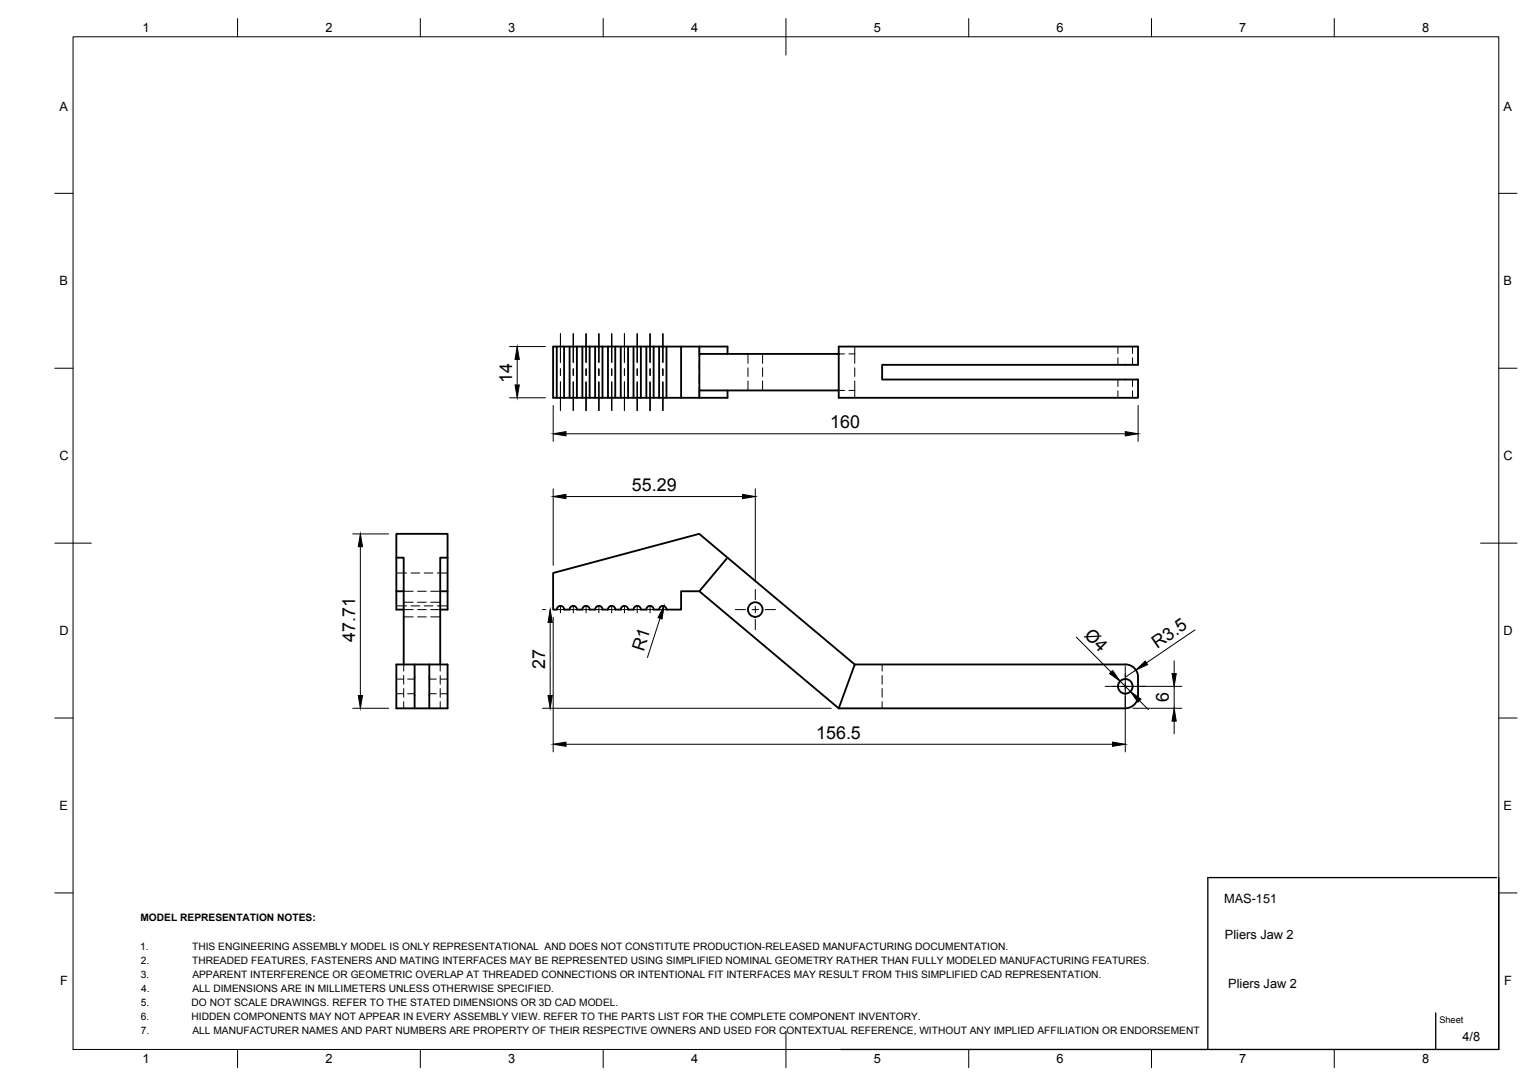
ISO-10303-21;
HEADER;
/* Generated by software containing ST-Developer
 * from STEP Tools, Inc. (www.steptools.com) 
 */

FILE_DESCRIPTION(
/* description */ ('STEP AP214'),
/* implementation_level */ '2;1');

FILE_NAME(
/* name */ 'Pliers Jaw 2.step',
/* time_stamp */ '2026-11-04T19:14:12-08:00',
/* author */ (''),
/* organization */ (''),
/* preprocessor_version */ 'ST-DEVELOPER v20.2',
/* originating_system */ 'Autodesk Translation Framework v15.17.0.0',
/* authorisation */ '');

FILE_SCHEMA (('AUTOMOTIVE_DESIGN { 1 0 10303 214 3 1 1 }'));
ENDSEC;

DATA;
#10=MECHANICAL_DESIGN_GEOMETRIC_PRESENTATION_REPRESENTATION('',(#100),#5990);
#86=SHAPE_REPRESENTATION_RELATIONSHIP('SRR','None',#6022,#93);
#93=ADVANCED_BREP_SHAPE_REPRESENTATION('',(#107),#5984);
#100=STYLED_ITEM('',(#6065),#107);
#107=MANIFOLD_SOLID_BREP('Body1',#3270);
#121=FACE_BOUND('',#479,.T.);
#122=FACE_BOUND('',#484,.T.);
#123=FACE_BOUND('',#516,.T.);
#124=FACE_BOUND('',#520,.T.);
#125=FACE_BOUND('',#522,.T.);
#126=FACE_BOUND('',#524,.T.);
#167=PLANE('',#3447);
#168=PLANE('',#3450);
#169=PLANE('',#3451);
#170=PLANE('',#3452);
#171=PLANE('',#3462);
#172=PLANE('',#3465);
#173=PLANE('',#3466);
#174=PLANE('',#3476);
#175=PLANE('',#3477);
#176=PLANE('',#3478);
#177=PLANE('',#3479);
#178=PLANE('',#3480);
#179=PLANE('',#3481);
#180=PLANE('',#3482);
#181=PLANE('',#3483);
#182=PLANE('',#3484);
#183=PLANE('',#3485);
#184=PLANE('',#3486);
#185=PLANE('',#3487);
#186=PLANE('',#3488);
#187=PLANE('',#3489);
#188=PLANE('',#3490);
#189=PLANE('',#3491);
#190=PLANE('',#3492);
#191=PLANE('',#3502);
#192=PLANE('',#3503);
#193=PLANE('',#3504);
#194=PLANE('',#3505);
#195=PLANE('',#3506);
#196=PLANE('',#3507);
#197=PLANE('',#3508);
#198=PLANE('',#3511);
#199=PLANE('',#3514);
#289=FACE_OUTER_BOUND('',#475,.T.);
#290=FACE_OUTER_BOUND('',#476,.T.);
#291=FACE_OUTER_BOUND('',#477,.T.);
#292=FACE_OUTER_BOUND('',#478,.T.);
#293=FACE_OUTER_BOUND('',#480,.T.);
#294=FACE_OUTER_BOUND('',#481,.T.);
#295=FACE_OUTER_BOUND('',#482,.T.);
#296=FACE_OUTER_BOUND('',#483,.T.);
#297=FACE_OUTER_BOUND('',#485,.T.);
#298=FACE_OUTER_BOUND('',#486,.T.);
#299=FACE_OUTER_BOUND('',#487,.T.);
#300=FACE_OUTER_BOUND('',#488,.T.);
#301=FACE_OUTER_BOUND('',#489,.T.);
#302=FACE_OUTER_BOUND('',#490,.T.);
#303=FACE_OUTER_BOUND('',#491,.T.);
#304=FACE_OUTER_BOUND('',#492,.T.);
#305=FACE_OUTER_BOUND('',#493,.T.);
#306=FACE_OUTER_BOUND('',#494,.T.);
#307=FACE_OUTER_BOUND('',#495,.T.);
#308=FACE_OUTER_BOUND('',#496,.T.);
#309=FACE_OUTER_BOUND('',#497,.T.);
#310=FACE_OUTER_BOUND('',#498,.T.);
#311=FACE_OUTER_BOUND('',#499,.T.);
#312=FACE_OUTER_BOUND('',#500,.T.);
#313=FACE_OUTER_BOUND('',#501,.T.);
#314=FACE_OUTER_BOUND('',#502,.T.);
#315=FACE_OUTER_BOUND('',#503,.T.);
#316=FACE_OUTER_BOUND('',#504,.T.);
#317=FACE_OUTER_BOUND('',#505,.T.);
#318=FACE_OUTER_BOUND('',#506,.T.);
#319=FACE_OUTER_BOUND('',#507,.T.);
#320=FACE_OUTER_BOUND('',#508,.T.);
#321=FACE_OUTER_BOUND('',#509,.T.);
#322=FACE_OUTER_BOUND('',#510,.T.);
#323=FACE_OUTER_BOUND('',#511,.T.);
#324=FACE_OUTER_BOUND('',#512,.T.);
#325=FACE_OUTER_BOUND('',#513,.T.);
#326=FACE_OUTER_BOUND('',#514,.T.);
#327=FACE_OUTER_BOUND('',#515,.T.);
#328=FACE_OUTER_BOUND('',#517,.T.);
#329=FACE_OUTER_BOUND('',#518,.T.);
#330=FACE_OUTER_BOUND('',#519,.T.);
#331=FACE_OUTER_BOUND('',#521,.T.);
#332=FACE_OUTER_BOUND('',#523,.T.);
#333=FACE_OUTER_BOUND('',#525,.T.);
#334=FACE_OUTER_BOUND('',#526,.T.);
#335=FACE_OUTER_BOUND('',#527,.T.);
#336=FACE_OUTER_BOUND('',#528,.T.);
#337=FACE_OUTER_BOUND('',#529,.T.);
#475=EDGE_LOOP('',(#2380,#2381,#2382,#2383));
#476=EDGE_LOOP('',(#2384,#2385,#2386,#2387));
#477=EDGE_LOOP('',(#2388,#2389,#2390,#2391));
#478=EDGE_LOOP('',(#2392,#2393,#2394,#2395,#2396,#2397));
#479=EDGE_LOOP('',(#2398));
#480=EDGE_LOOP('',(#2399,#2400,#2401,#2402));
#481=EDGE_LOOP('',(#2403,#2404,#2405,#2406,#2407,#2408,#2409,#2410));
#482=EDGE_LOOP('',(#2411,#2412,#2413,#2414,#2415,#2416,#2417,#2418,#2419,
#2420,#2421,#2422,#2423,#2424,#2425,#2426,#2427,#2428,#2429,#2430,#2431,
#2432,#2433,#2434,#2435));
#483=EDGE_LOOP('',(#2436,#2437,#2438,#2439,#2440,#2441));
#484=EDGE_LOOP('',(#2442));
#485=EDGE_LOOP('',(#2443,#2444,#2445,#2446));
#486=EDGE_LOOP('',(#2447,#2448,#2449,#2450,#2451,#2452,#2453,#2454,#2455,
#2456,#2457,#2458,#2459,#2460,#2461,#2462,#2463,#2464,#2465,#2466,#2467,
#2468,#2469,#2470,#2471));
#487=EDGE_LOOP('',(#2472,#2473,#2474,#2475));
#488=EDGE_LOOP('',(#2476,#2477,#2478,#2479));
#489=EDGE_LOOP('',(#2480,#2481,#2482,#2483));
#490=EDGE_LOOP('',(#2484,#2485,#2486,#2487));
#491=EDGE_LOOP('',(#2488,#2489,#2490,#2491));
#492=EDGE_LOOP('',(#2492,#2493,#2494,#2495));
#493=EDGE_LOOP('',(#2496,#2497,#2498,#2499));
#494=EDGE_LOOP('',(#2500,#2501,#2502,#2503));
#495=EDGE_LOOP('',(#2504,#2505,#2506,#2507));
#496=EDGE_LOOP('',(#2508,#2509,#2510,#2511,#2512,#2513));
#497=EDGE_LOOP('',(#2514,#2515,#2516,#2517));
#498=EDGE_LOOP('',(#2518,#2519,#2520,#2521));
#499=EDGE_LOOP('',(#2522,#2523,#2524,#2525,#2526,#2527,#2528,#2529,#2530,
#2531));
#500=EDGE_LOOP('',(#2532,#2533,#2534,#2535));
#501=EDGE_LOOP('',(#2536,#2537,#2538,#2539,#2540,#2541,#2542,#2543,#2544,
#2545));
#502=EDGE_LOOP('',(#2546,#2547,#2548,#2549));
#503=EDGE_LOOP('',(#2550,#2551,#2552,#2553));
#504=EDGE_LOOP('',(#2554,#2555,#2556,#2557));
#505=EDGE_LOOP('',(#2558,#2559,#2560,#2561));
#506=EDGE_LOOP('',(#2562,#2563,#2564,#2565));
#507=EDGE_LOOP('',(#2566,#2567,#2568,#2569));
#508=EDGE_LOOP('',(#2570,#2571,#2572,#2573));
#509=EDGE_LOOP('',(#2574,#2575,#2576,#2577));
#510=EDGE_LOOP('',(#2578,#2579,#2580,#2581));
#511=EDGE_LOOP('',(#2582,#2583,#2584,#2585));
#512=EDGE_LOOP('',(#2586,#2587,#2588,#2589));
#513=EDGE_LOOP('',(#2590,#2591,#2592,#2593));
#514=EDGE_LOOP('',(#2594,#2595,#2596,#2597));
#515=EDGE_LOOP('',(#2598,#2599,#2600,#2601));
#516=EDGE_LOOP('',(#2602));
#517=EDGE_LOOP('',(#2603,#2604,#2605,#2606));
#518=EDGE_LOOP('',(#2607,#2608,#2609,#2610));
#519=EDGE_LOOP('',(#2611,#2612,#2613,#2614));
#520=EDGE_LOOP('',(#2615));
#521=EDGE_LOOP('',(#2616,#2617,#2618,#2619,#2620,#2621));
#522=EDGE_LOOP('',(#2622));
#523=EDGE_LOOP('',(#2623,#2624,#2625,#2626,#2627,#2628));
#524=EDGE_LOOP('',(#2629));
#525=EDGE_LOOP('',(#2630,#2631,#2632,#2633));
#526=EDGE_LOOP('',(#2634,#2635,#2636,#2637));
#527=EDGE_LOOP('',(#2638,#2639,#2640,#2641));
#528=EDGE_LOOP('',(#2642,#2643,#2644,#2645));
#529=EDGE_LOOP('',(#2646,#2647,#2648,#2649));
#723=LINE('',#4927,#1026);
#724=LINE('',#4933,#1027);
#725=LINE('',#4939,#1028);
#726=LINE('',#4944,#1029);
#727=LINE('',#4948,#1030);
#728=LINE('',#4952,#1031);
#729=LINE('',#4953,#1032);
#730=LINE('',#4956,#1033);
#731=LINE('',#4958,#1034);
#732=LINE('',#4959,#1035);
#733=LINE('',#4963,#1036);
#734=LINE('',#4965,#1037);
#735=LINE('',#4967,#1038);
#736=LINE('',#4969,#1039);
#737=LINE('',#4971,#1040);
#738=LINE('',#4973,#1041);
#739=LINE('',#4975,#1042);
#740=LINE('',#4976,#1043);
#741=LINE('',#4979,#1044);
#742=LINE('',#4981,#1045);
#743=LINE('',#4983,#1046);
#744=LINE('',#4985,#1047);
#745=LINE('',#4989,#1048);
#746=LINE('',#4993,#1049);
#747=LINE('',#4997,#1050);
#748=LINE('',#5001,#1051);
#749=LINE('',#5005,#1052);
#750=LINE('',#5009,#1053);
#751=LINE('',#5013,#1054);
#752=LINE('',#5017,#1055);
#753=LINE('',#5021,#1056);
#754=LINE('',#5023,#1057);
#755=LINE('',#5024,#1058);
#756=LINE('',#5028,#1059);
#757=LINE('',#5032,#1060);
#758=LINE('',#5034,#1061);
#759=LINE('',#5036,#1062);
#760=LINE('',#5041,#1063);
#761=LINE('',#5043,#1064);
#762=LINE('',#5045,#1065);
#763=LINE('',#5046,#1066);
#764=LINE('',#5049,#1067);
#765=LINE('',#5051,#1068);
#766=LINE('',#5053,#1069);
#767=LINE('',#5055,#1070);
#768=LINE('',#5059,#1071);
#769=LINE('',#5063,#1072);
#770=LINE('',#5067,#1073);
#771=LINE('',#5071,#1074);
#772=LINE('',#5075,#1075);
#773=LINE('',#5079,#1076);
#774=LINE('',#5083,#1077);
#775=LINE('',#5087,#1078);
#776=LINE('',#5091,#1079);
#777=LINE('',#5093,#1080);
#778=LINE('',#5094,#1081);
#779=LINE('',#5096,#1082);
#780=LINE('',#5097,#1083);
#781=LINE('',#5099,#1084);
#782=LINE('',#5100,#1085);
#783=LINE('',#5102,#1086);
#784=LINE('',#5103,#1087);
#785=LINE('',#5105,#1088);
#786=LINE('',#5106,#1089);
#787=LINE('',#5108,#1090);
#788=LINE('',#5109,#1091);
#789=LINE('',#5111,#1092);
#790=LINE('',#5112,#1093);
#791=LINE('',#5114,#1094);
#792=LINE('',#5115,#1095);
#793=LINE('',#5117,#1096);
#794=LINE('',#5118,#1097);
#795=LINE('',#5120,#1098);
#796=LINE('',#5121,#1099);
#797=LINE('',#5123,#1100);
#798=LINE('',#5124,#1101);
#799=LINE('',#5125,#1102);
#800=LINE('',#5127,#1103);
#801=LINE('',#5128,#1104);
#802=LINE('',#5132,#1105);
#803=LINE('',#5134,#1106);
#804=LINE('',#5136,#1107);
#805=LINE('',#5138,#1108);
#806=LINE('',#5139,#1109);
#807=LINE('',#5140,#1110);
#808=LINE('',#5141,#1111);
#809=LINE('',#5145,#1112);
#810=LINE('',#5146,#1113);
#811=LINE('',#5147,#1114);
#812=LINE('',#5150,#1115);
#813=LINE('',#5152,#1116);
#814=LINE('',#5154,#1117);
#815=LINE('',#5156,#1118);
#816=LINE('',#5157,#1119);
#817=LINE('',#5158,#1120);
#818=LINE('',#5159,#1121);
#819=LINE('',#5162,#1122);
#820=LINE('',#5173,#1123);
#821=LINE('',#5175,#1124);
#822=LINE('',#5178,#1125);
#823=LINE('',#5180,#1126);
#824=LINE('',#5185,#1127);
#825=LINE('',#5188,#1128);
#1026=VECTOR('',#3958,2.);
#1027=VECTOR('',#3965,2.);
#1028=VECTOR('',#3972,2.);
#1029=VECTOR('',#3977,1000.);
#1030=VECTOR('',#3980,1000.);
#1031=VECTOR('',#3983,1000.);
#1032=VECTOR('',#3984,1000.);
#1033=VECTOR('',#3987,1000.);
#1034=VECTOR('',#3988,1000.);
#1035=VECTOR('',#3989,1000.);
#1036=VECTOR('',#3992,1000.);
#1037=VECTOR('',#3993,1000.);
#1038=VECTOR('',#3994,1000.);
#1039=VECTOR('',#3995,1000.);
#1040=VECTOR('',#3996,1000.);
#1041=VECTOR('',#3997,1000.);
#1042=VECTOR('',#3998,1000.);
#1043=VECTOR('',#3999,1000.);
#1044=VECTOR('',#4002,1000.);
#1045=VECTOR('',#4003,1000.);
#1046=VECTOR('',#4004,1000.);
#1047=VECTOR('',#4005,1000.);
#1048=VECTOR('',#4008,1000.);
#1049=VECTOR('',#4011,1000.);
#1050=VECTOR('',#4014,1000.);
#1051=VECTOR('',#4017,1000.);
#1052=VECTOR('',#4020,1000.);
#1053=VECTOR('',#4023,1000.);
#1054=VECTOR('',#4026,1000.);
#1055=VECTOR('',#4029,1000.);
#1056=VECTOR('',#4032,1000.);
#1057=VECTOR('',#4033,1000.);
#1058=VECTOR('',#4034,1000.);
#1059=VECTOR('',#4037,1000.);
#1060=VECTOR('',#4040,1000.);
#1061=VECTOR('',#4041,1000.);
#1062=VECTOR('',#4042,1000.);
#1063=VECTOR('',#4047,1000.);
#1064=VECTOR('',#4048,1000.);
#1065=VECTOR('',#4049,1000.);
#1066=VECTOR('',#4050,1000.);
#1067=VECTOR('',#4053,1000.);
#1068=VECTOR('',#4054,1000.);
#1069=VECTOR('',#4055,1000.);
#1070=VECTOR('',#4056,1000.);
#1071=VECTOR('',#4059,1000.);
#1072=VECTOR('',#4062,1000.);
#1073=VECTOR('',#4065,1000.);
#1074=VECTOR('',#4068,1000.);
#1075=VECTOR('',#4071,1000.);
#1076=VECTOR('',#4074,1000.);
#1077=VECTOR('',#4077,1000.);
#1078=VECTOR('',#4080,1000.);
#1079=VECTOR('',#4083,1000.);
#1080=VECTOR('',#4084,1000.);
#1081=VECTOR('',#4085,1000.);
#1082=VECTOR('',#4088,1000.);
#1083=VECTOR('',#4089,1000.);
#1084=VECTOR('',#4092,1000.);
#1085=VECTOR('',#4093,1000.);
#1086=VECTOR('',#4096,1000.);
#1087=VECTOR('',#4097,1000.);
#1088=VECTOR('',#4100,1000.);
#1089=VECTOR('',#4101,1000.);
#1090=VECTOR('',#4104,1000.);
#1091=VECTOR('',#4105,1000.);
#1092=VECTOR('',#4108,1000.);
#1093=VECTOR('',#4109,1000.);
#1094=VECTOR('',#4112,1000.);
#1095=VECTOR('',#4113,1000.);
#1096=VECTOR('',#4116,1000.);
#1097=VECTOR('',#4117,1000.);
#1098=VECTOR('',#4120,1000.);
#1099=VECTOR('',#4121,1000.);
#1100=VECTOR('',#4124,1000.);
#1101=VECTOR('',#4125,1000.);
#1102=VECTOR('',#4126,1000.);
#1103=VECTOR('',#4129,1000.);
#1104=VECTOR('',#4130,1000.);
#1105=VECTOR('',#4135,1000.);
#1106=VECTOR('',#4136,1000.);
#1107=VECTOR('',#4137,1000.);
#1108=VECTOR('',#4138,1000.);
#1109=VECTOR('',#4139,1000.);
#1110=VECTOR('',#4140,1000.);
#1111=VECTOR('',#4141,1000.);
#1112=VECTOR('',#4144,1000.);
#1113=VECTOR('',#4145,1000.);
#1114=VECTOR('',#4146,1000.);
#1115=VECTOR('',#4149,1000.);
#1116=VECTOR('',#4150,1000.);
#1117=VECTOR('',#4151,1000.);
#1118=VECTOR('',#4152,1000.);
#1119=VECTOR('',#4153,1000.);
#1120=VECTOR('',#4154,1000.);
#1121=VECTOR('',#4155,1000.);
#1122=VECTOR('',#4160,1000.);
#1123=VECTOR('',#4181,1000.);
#1124=VECTOR('',#4184,1000.);
#1125=VECTOR('',#4189,1000.);
#1126=VECTOR('',#4192,1000.);
#1127=VECTOR('',#4201,1000.);
#1128=VECTOR('',#4206,1000.);
#1262=CIRCLE('',#3439,2.);
#1263=CIRCLE('',#3440,2.);
#1264=CIRCLE('',#3442,2.);
#1265=CIRCLE('',#3443,2.);
#1266=CIRCLE('',#3445,2.);
#1267=CIRCLE('',#3446,2.);
#1268=CIRCLE('',#3448,3.5);
#1269=CIRCLE('',#3449,3.5);
#1270=CIRCLE('',#3453,1.);
#1271=CIRCLE('',#3454,1.);
#1272=CIRCLE('',#3455,1.);
#1273=CIRCLE('',#3456,1.);
#1274=CIRCLE('',#3457,1.);
#1275=CIRCLE('',#3458,1.);
#1276=CIRCLE('',#3459,1.);
#1277=CIRCLE('',#3460,1.);
#1278=CIRCLE('',#3461,1.);
#1279=CIRCLE('',#3463,3.5);
#1280=CIRCLE('',#3464,3.5);
#1281=CIRCLE('',#3467,1.);
#1282=CIRCLE('',#3468,1.);
#1283=CIRCLE('',#3469,1.);
#1284=CIRCLE('',#3470,1.);
#1285=CIRCLE('',#3471,1.);
#1286=CIRCLE('',#3472,1.);
#1287=CIRCLE('',#3473,1.);
#1288=CIRCLE('',#3474,1.);
#1289=CIRCLE('',#3475,1.);
#1290=CIRCLE('',#3509,3.5);
#1291=CIRCLE('',#3510,3.5);
#1292=CIRCLE('',#3512,3.5);
#1293=CIRCLE('',#3513,3.5);
#1444=VERTEX_POINT('',#4924);
#1445=VERTEX_POINT('',#4926);
#1446=VERTEX_POINT('',#4930);
#1447=VERTEX_POINT('',#4932);
#1448=VERTEX_POINT('',#4936);
#1449=VERTEX_POINT('',#4938);
#1450=VERTEX_POINT('',#4942);
#1451=VERTEX_POINT('',#4943);
#1452=VERTEX_POINT('',#4945);
#1453=VERTEX_POINT('',#4947);
#1454=VERTEX_POINT('',#4949);
#1455=VERTEX_POINT('',#4951);
#1456=VERTEX_POINT('',#4955);
#1457=VERTEX_POINT('',#4957);
#1458=VERTEX_POINT('',#4961);
#1459=VERTEX_POINT('',#4962);
#1460=VERTEX_POINT('',#4964);
#1461=VERTEX_POINT('',#4966);
#1462=VERTEX_POINT('',#4968);
#1463=VERTEX_POINT('',#4970);
#1464=VERTEX_POINT('',#4972);
#1465=VERTEX_POINT('',#4974);
#1466=VERTEX_POINT('',#4978);
#1467=VERTEX_POINT('',#4980);
#1468=VERTEX_POINT('',#4982);
#1469=VERTEX_POINT('',#4984);
#1470=VERTEX_POINT('',#4986);
#1471=VERTEX_POINT('',#4988);
#1472=VERTEX_POINT('',#4990);
#1473=VERTEX_POINT('',#4992);
#1474=VERTEX_POINT('',#4994);
#1475=VERTEX_POINT('',#4996);
#1476=VERTEX_POINT('',#4998);
#1477=VERTEX_POINT('',#5000);
#1478=VERTEX_POINT('',#5002);
#1479=VERTEX_POINT('',#5004);
#1480=VERTEX_POINT('',#5006);
#1481=VERTEX_POINT('',#5008);
#1482=VERTEX_POINT('',#5010);
#1483=VERTEX_POINT('',#5012);
#1484=VERTEX_POINT('',#5014);
#1485=VERTEX_POINT('',#5016);
#1486=VERTEX_POINT('',#5018);
#1487=VERTEX_POINT('',#5020);
#1488=VERTEX_POINT('',#5022);
#1489=VERTEX_POINT('',#5026);
#1490=VERTEX_POINT('',#5027);
#1491=VERTEX_POINT('',#5029);
#1492=VERTEX_POINT('',#5031);
#1493=VERTEX_POINT('',#5033);
#1494=VERTEX_POINT('',#5035);
#1495=VERTEX_POINT('',#5039);
#1496=VERTEX_POINT('',#5040);
#1497=VERTEX_POINT('',#5042);
#1498=VERTEX_POINT('',#5044);
#1499=VERTEX_POINT('',#5048);
#1500=VERTEX_POINT('',#5050);
#1501=VERTEX_POINT('',#5052);
#1502=VERTEX_POINT('',#5054);
#1503=VERTEX_POINT('',#5056);
#1504=VERTEX_POINT('',#5058);
#1505=VERTEX_POINT('',#5060);
#1506=VERTEX_POINT('',#5062);
#1507=VERTEX_POINT('',#5064);
#1508=VERTEX_POINT('',#5066);
#1509=VERTEX_POINT('',#5068);
#1510=VERTEX_POINT('',#5070);
#1511=VERTEX_POINT('',#5072);
#1512=VERTEX_POINT('',#5074);
#1513=VERTEX_POINT('',#5076);
#1514=VERTEX_POINT('',#5078);
#1515=VERTEX_POINT('',#5080);
#1516=VERTEX_POINT('',#5082);
#1517=VERTEX_POINT('',#5084);
#1518=VERTEX_POINT('',#5086);
#1519=VERTEX_POINT('',#5088);
#1520=VERTEX_POINT('',#5090);
#1521=VERTEX_POINT('',#5092);
#1522=VERTEX_POINT('',#5131);
#1523=VERTEX_POINT('',#5133);
#1524=VERTEX_POINT('',#5135);
#1525=VERTEX_POINT('',#5137);
#1526=VERTEX_POINT('',#5143);
#1527=VERTEX_POINT('',#5144);
#1528=VERTEX_POINT('',#5149);
#1529=VERTEX_POINT('',#5151);
#1530=VERTEX_POINT('',#5153);
#1531=VERTEX_POINT('',#5155);
#1786=EDGE_CURVE('',#1444,#1444,#1262,.T.);
#1787=EDGE_CURVE('',#1444,#1445,#723,.T.);
#1788=EDGE_CURVE('',#1445,#1445,#1263,.T.);
#1789=EDGE_CURVE('',#1446,#1446,#1264,.T.);
#1790=EDGE_CURVE('',#1446,#1447,#724,.T.);
#1791=EDGE_CURVE('',#1447,#1447,#1265,.T.);
#1792=EDGE_CURVE('',#1448,#1448,#1266,.T.);
#1793=EDGE_CURVE('',#1448,#1449,#725,.T.);
#1794=EDGE_CURVE('',#1449,#1449,#1267,.T.);
#1795=EDGE_CURVE('',#1450,#1451,#726,.T.);
#1796=EDGE_CURVE('',#1451,#1452,#1268,.T.);
#1797=EDGE_CURVE('',#1452,#1453,#727,.T.);
#1798=EDGE_CURVE('',#1453,#1454,#1269,.T.);
#1799=EDGE_CURVE('',#1454,#1455,#728,.T.);
#1800=EDGE_CURVE('',#1455,#1450,#729,.T.);
#1801=EDGE_CURVE('',#1452,#1456,#730,.T.);
#1802=EDGE_CURVE('',#1456,#1457,#731,.T.);
#1803=EDGE_CURVE('',#1457,#1453,#732,.T.);
#1804=EDGE_CURVE('',#1458,#1459,#733,.T.);
#1805=EDGE_CURVE('',#1460,#1458,#734,.T.);
#1806=EDGE_CURVE('',#1460,#1461,#735,.T.);
#1807=EDGE_CURVE('',#1461,#1462,#736,.T.);
#1808=EDGE_CURVE('',#1462,#1463,#737,.T.);
#1809=EDGE_CURVE('',#1464,#1463,#738,.T.);
#1810=EDGE_CURVE('',#1465,#1464,#739,.T.);
#1811=EDGE_CURVE('',#1465,#1459,#740,.T.);
#1812=EDGE_CURVE('',#1458,#1466,#741,.T.);
#1813=EDGE_CURVE('',#1466,#1467,#742,.T.);
#1814=EDGE_CURVE('',#1467,#1468,#743,.T.);
#1815=EDGE_CURVE('',#1468,#1469,#744,.T.);
#1816=EDGE_CURVE('',#1470,#1469,#1270,.T.);
#1817=EDGE_CURVE('',#1470,#1471,#745,.T.);
#1818=EDGE_CURVE('',#1472,#1471,#1271,.T.);
#1819=EDGE_CURVE('',#1472,#1473,#746,.T.);
#1820=EDGE_CURVE('',#1474,#1473,#1272,.T.);
#1821=EDGE_CURVE('',#1474,#1475,#747,.T.);
#1822=EDGE_CURVE('',#1476,#1475,#1273,.T.);
#1823=EDGE_CURVE('',#1476,#1477,#748,.T.);
#1824=EDGE_CURVE('',#1478,#1477,#1274,.T.);
#1825=EDGE_CURVE('',#1478,#1479,#749,.T.);
#1826=EDGE_CURVE('',#1480,#1479,#1275,.T.);
#1827=EDGE_CURVE('',#1480,#1481,#750,.T.);
#1828=EDGE_CURVE('',#1482,#1481,#1276,.T.);
#1829=EDGE_CURVE('',#1482,#1483,#751,.T.);
#1830=EDGE_CURVE('',#1484,#1483,#1277,.T.);
#1831=EDGE_CURVE('',#1484,#1485,#752,.T.);
#1832=EDGE_CURVE('',#1486,#1485,#1278,.T.);
#1833=EDGE_CURVE('',#1486,#1487,#753,.T.);
#1834=EDGE_CURVE('',#1487,#1488,#754,.T.);
#1835=EDGE_CURVE('',#1488,#1460,#755,.T.);
#1836=EDGE_CURVE('',#1489,#1490,#756,.T.);
#1837=EDGE_CURVE('',#1489,#1491,#1279,.T.);
#1838=EDGE_CURVE('',#1492,#1491,#757,.T.);
#1839=EDGE_CURVE('',#1493,#1492,#758,.T.);
#1840=EDGE_CURVE('',#1494,#1493,#759,.T.);
#1841=EDGE_CURVE('',#1494,#1490,#1280,.T.);
#1842=EDGE_CURVE('',#1495,#1496,#760,.T.);
#1843=EDGE_CURVE('',#1495,#1497,#761,.T.);
#1844=EDGE_CURVE('',#1497,#1498,#762,.T.);
#1845=EDGE_CURVE('',#1496,#1498,#763,.T.);
#1846=EDGE_CURVE('',#1462,#1499,#764,.T.);
#1847=EDGE_CURVE('',#1500,#1461,#765,.T.);
#1848=EDGE_CURVE('',#1501,#1500,#766,.T.);
#1849=EDGE_CURVE('',#1502,#1501,#767,.T.);
#1850=EDGE_CURVE('',#1502,#1503,#1281,.T.);
#1851=EDGE_CURVE('',#1504,#1503,#768,.T.);
#1852=EDGE_CURVE('',#1504,#1505,#1282,.T.);
#1853=EDGE_CURVE('',#1506,#1505,#769,.T.);
#1854=EDGE_CURVE('',#1506,#1507,#1283,.T.);
#1855=EDGE_CURVE('',#1508,#1507,#770,.T.);
#1856=EDGE_CURVE('',#1508,#1509,#1284,.T.);
#1857=EDGE_CURVE('',#1510,#1509,#771,.T.);
#1858=EDGE_CURVE('',#1510,#1511,#1285,.T.);
#1859=EDGE_CURVE('',#1512,#1511,#772,.T.);
#1860=EDGE_CURVE('',#1512,#1513,#1286,.T.);
#1861=EDGE_CURVE('',#1514,#1513,#773,.T.);
#1862=EDGE_CURVE('',#1514,#1515,#1287,.T.);
#1863=EDGE_CURVE('',#1516,#1515,#774,.T.);
#1864=EDGE_CURVE('',#1516,#1517,#1288,.T.);
#1865=EDGE_CURVE('',#1518,#1517,#775,.T.);
#1866=EDGE_CURVE('',#1518,#1519,#1289,.T.);
#1867=EDGE_CURVE('',#1520,#1519,#776,.T.);
#1868=EDGE_CURVE('',#1521,#1520,#777,.T.);
#1869=EDGE_CURVE('',#1499,#1521,#778,.T.);
#1870=EDGE_CURVE('',#1505,#1483,#779,.T.);
#1871=EDGE_CURVE('',#1482,#1506,#780,.T.);
#1872=EDGE_CURVE('',#1507,#1481,#781,.T.);
#1873=EDGE_CURVE('',#1480,#1508,#782,.T.);
#1874=EDGE_CURVE('',#1509,#1479,#783,.T.);
#1875=EDGE_CURVE('',#1478,#1510,#784,.T.);
#1876=EDGE_CURVE('',#1511,#1477,#785,.T.);
#1877=EDGE_CURVE('',#1476,#1512,#786,.T.);
#1878=EDGE_CURVE('',#1513,#1475,#787,.T.);
#1879=EDGE_CURVE('',#1474,#1514,#788,.T.);
#1880=EDGE_CURVE('',#1515,#1473,#789,.T.);
#1881=EDGE_CURVE('',#1472,#1516,#790,.T.);
#1882=EDGE_CURVE('',#1517,#1471,#791,.T.);
#1883=EDGE_CURVE('',#1470,#1518,#792,.T.);
#1884=EDGE_CURVE('',#1519,#1469,#793,.T.);
#1885=EDGE_CURVE('',#1468,#1520,#794,.T.);
#1886=EDGE_CURVE('',#1484,#1504,#795,.T.);
#1887=EDGE_CURVE('',#1503,#1485,#796,.T.);
#1888=EDGE_CURVE('',#1467,#1521,#797,.T.);
#1889=EDGE_CURVE('',#1466,#1495,#798,.T.);
#1890=EDGE_CURVE('',#1499,#1496,#799,.T.);
#1891=EDGE_CURVE('',#1488,#1500,#800,.T.);
#1892=EDGE_CURVE('',#1487,#1501,#801,.T.);
#1893=EDGE_CURVE('',#1491,#1522,#802,.T.);
#1894=EDGE_CURVE('',#1522,#1523,#803,.T.);
#1895=EDGE_CURVE('',#1524,#1523,#804,.T.);
#1896=EDGE_CURVE('',#1525,#1524,#805,.T.);
#1897=EDGE_CURVE('',#1525,#1451,#806,.T.);
#1898=EDGE_CURVE('',#1450,#1465,#807,.T.);
#1899=EDGE_CURVE('',#1492,#1464,#808,.T.);
#1900=EDGE_CURVE('',#1526,#1527,#809,.T.);
#1901=EDGE_CURVE('',#1526,#1489,#810,.T.);
#1902=EDGE_CURVE('',#1490,#1527,#811,.T.);
#1903=EDGE_CURVE('',#1454,#1528,#812,.T.);
#1904=EDGE_CURVE('',#1528,#1529,#813,.T.);
#1905=EDGE_CURVE('',#1529,#1530,#814,.T.);
#1906=EDGE_CURVE('',#1531,#1530,#815,.T.);
#1907=EDGE_CURVE('',#1531,#1494,#816,.T.);
#1908=EDGE_CURVE('',#1493,#1498,#817,.T.);
#1909=EDGE_CURVE('',#1455,#1497,#818,.T.);
#1910=EDGE_CURVE('',#1486,#1502,#819,.T.);
#1911=EDGE_CURVE('',#1498,#1464,#820,.T.);
#1912=EDGE_CURVE('',#1463,#1496,#821,.T.);
#1913=EDGE_CURVE('',#1497,#1465,#822,.T.);
#1914=EDGE_CURVE('',#1459,#1495,#823,.T.);
#1915=EDGE_CURVE('',#1522,#1526,#1290,.T.);
#1916=EDGE_CURVE('',#1527,#1531,#1291,.T.);
#1917=EDGE_CURVE('',#1523,#1530,#824,.T.);
#1918=EDGE_CURVE('',#1456,#1525,#1292,.T.);
#1919=EDGE_CURVE('',#1524,#1529,#825,.T.);
#1920=EDGE_CURVE('',#1528,#1457,#1293,.T.);
#2380=ORIENTED_EDGE('',*,*,#1786,.F.);
#2381=ORIENTED_EDGE('',*,*,#1787,.T.);
#2382=ORIENTED_EDGE('',*,*,#1788,.F.);
#2383=ORIENTED_EDGE('',*,*,#1787,.F.);
#2384=ORIENTED_EDGE('',*,*,#1789,.T.);
#2385=ORIENTED_EDGE('',*,*,#1790,.T.);
#2386=ORIENTED_EDGE('',*,*,#1791,.T.);
#2387=ORIENTED_EDGE('',*,*,#1790,.F.);
#2388=ORIENTED_EDGE('',*,*,#1792,.F.);
#2389=ORIENTED_EDGE('',*,*,#1793,.T.);
#2390=ORIENTED_EDGE('',*,*,#1794,.F.);
#2391=ORIENTED_EDGE('',*,*,#1793,.F.);
#2392=ORIENTED_EDGE('',*,*,#1795,.T.);
#2393=ORIENTED_EDGE('',*,*,#1796,.T.);
#2394=ORIENTED_EDGE('',*,*,#1797,.T.);
#2395=ORIENTED_EDGE('',*,*,#1798,.T.);
#2396=ORIENTED_EDGE('',*,*,#1799,.T.);
#2397=ORIENTED_EDGE('',*,*,#1800,.T.);
#2398=ORIENTED_EDGE('',*,*,#1791,.F.);
#2399=ORIENTED_EDGE('',*,*,#1797,.F.);
#2400=ORIENTED_EDGE('',*,*,#1801,.T.);
#2401=ORIENTED_EDGE('',*,*,#1802,.T.);
#2402=ORIENTED_EDGE('',*,*,#1803,.T.);
#2403=ORIENTED_EDGE('',*,*,#1804,.F.);
#2404=ORIENTED_EDGE('',*,*,#1805,.F.);
#2405=ORIENTED_EDGE('',*,*,#1806,.T.);
#2406=ORIENTED_EDGE('',*,*,#1807,.T.);
#2407=ORIENTED_EDGE('',*,*,#1808,.T.);
#2408=ORIENTED_EDGE('',*,*,#1809,.F.);
#2409=ORIENTED_EDGE('',*,*,#1810,.F.);
#2410=ORIENTED_EDGE('',*,*,#1811,.T.);
#2411=ORIENTED_EDGE('',*,*,#1812,.T.);
#2412=ORIENTED_EDGE('',*,*,#1813,.T.);
#2413=ORIENTED_EDGE('',*,*,#1814,.T.);
#2414=ORIENTED_EDGE('',*,*,#1815,.T.);
#2415=ORIENTED_EDGE('',*,*,#1816,.F.);
#2416=ORIENTED_EDGE('',*,*,#1817,.T.);
#2417=ORIENTED_EDGE('',*,*,#1818,.F.);
#2418=ORIENTED_EDGE('',*,*,#1819,.T.);
#2419=ORIENTED_EDGE('',*,*,#1820,.F.);
#2420=ORIENTED_EDGE('',*,*,#1821,.T.);
#2421=ORIENTED_EDGE('',*,*,#1822,.F.);
#2422=ORIENTED_EDGE('',*,*,#1823,.T.);
#2423=ORIENTED_EDGE('',*,*,#1824,.F.);
#2424=ORIENTED_EDGE('',*,*,#1825,.T.);
#2425=ORIENTED_EDGE('',*,*,#1826,.F.);
#2426=ORIENTED_EDGE('',*,*,#1827,.T.);
#2427=ORIENTED_EDGE('',*,*,#1828,.F.);
#2428=ORIENTED_EDGE('',*,*,#1829,.T.);
#2429=ORIENTED_EDGE('',*,*,#1830,.F.);
#2430=ORIENTED_EDGE('',*,*,#1831,.T.);
#2431=ORIENTED_EDGE('',*,*,#1832,.F.);
#2432=ORIENTED_EDGE('',*,*,#1833,.T.);
#2433=ORIENTED_EDGE('',*,*,#1834,.T.);
#2434=ORIENTED_EDGE('',*,*,#1835,.T.);
#2435=ORIENTED_EDGE('',*,*,#1805,.T.);
#2436=ORIENTED_EDGE('',*,*,#1836,.F.);
#2437=ORIENTED_EDGE('',*,*,#1837,.T.);
#2438=ORIENTED_EDGE('',*,*,#1838,.F.);
#2439=ORIENTED_EDGE('',*,*,#1839,.F.);
#2440=ORIENTED_EDGE('',*,*,#1840,.F.);
#2441=ORIENTED_EDGE('',*,*,#1841,.T.);
#2442=ORIENTED_EDGE('',*,*,#1786,.T.);
#2443=ORIENTED_EDGE('',*,*,#1842,.F.);
#2444=ORIENTED_EDGE('',*,*,#1843,.T.);
#2445=ORIENTED_EDGE('',*,*,#1844,.T.);
#2446=ORIENTED_EDGE('',*,*,#1845,.F.);
#2447=ORIENTED_EDGE('',*,*,#1846,.F.);
#2448=ORIENTED_EDGE('',*,*,#1807,.F.);
#2449=ORIENTED_EDGE('',*,*,#1847,.F.);
#2450=ORIENTED_EDGE('',*,*,#1848,.F.);
#2451=ORIENTED_EDGE('',*,*,#1849,.F.);
#2452=ORIENTED_EDGE('',*,*,#1850,.T.);
#2453=ORIENTED_EDGE('',*,*,#1851,.F.);
#2454=ORIENTED_EDGE('',*,*,#1852,.T.);
#2455=ORIENTED_EDGE('',*,*,#1853,.F.);
#2456=ORIENTED_EDGE('',*,*,#1854,.T.);
#2457=ORIENTED_EDGE('',*,*,#1855,.F.);
#2458=ORIENTED_EDGE('',*,*,#1856,.T.);
#2459=ORIENTED_EDGE('',*,*,#1857,.F.);
#2460=ORIENTED_EDGE('',*,*,#1858,.T.);
#2461=ORIENTED_EDGE('',*,*,#1859,.F.);
#2462=ORIENTED_EDGE('',*,*,#1860,.T.);
#2463=ORIENTED_EDGE('',*,*,#1861,.F.);
#2464=ORIENTED_EDGE('',*,*,#1862,.T.);
#2465=ORIENTED_EDGE('',*,*,#1863,.F.);
#2466=ORIENTED_EDGE('',*,*,#1864,.T.);
#2467=ORIENTED_EDGE('',*,*,#1865,.F.);
#2468=ORIENTED_EDGE('',*,*,#1866,.T.);
#2469=ORIENTED_EDGE('',*,*,#1867,.F.);
#2470=ORIENTED_EDGE('',*,*,#1868,.F.);
#2471=ORIENTED_EDGE('',*,*,#1869,.F.);
#2472=ORIENTED_EDGE('',*,*,#1853,.T.);
#2473=ORIENTED_EDGE('',*,*,#1870,.T.);
#2474=ORIENTED_EDGE('',*,*,#1829,.F.);
#2475=ORIENTED_EDGE('',*,*,#1871,.T.);
#2476=ORIENTED_EDGE('',*,*,#1855,.T.);
#2477=ORIENTED_EDGE('',*,*,#1872,.T.);
#2478=ORIENTED_EDGE('',*,*,#1827,.F.);
#2479=ORIENTED_EDGE('',*,*,#1873,.T.);
#2480=ORIENTED_EDGE('',*,*,#1857,.T.);
#2481=ORIENTED_EDGE('',*,*,#1874,.T.);
#2482=ORIENTED_EDGE('',*,*,#1825,.F.);
#2483=ORIENTED_EDGE('',*,*,#1875,.T.);
#2484=ORIENTED_EDGE('',*,*,#1859,.T.);
#2485=ORIENTED_EDGE('',*,*,#1876,.T.);
#2486=ORIENTED_EDGE('',*,*,#1823,.F.);
#2487=ORIENTED_EDGE('',*,*,#1877,.T.);
#2488=ORIENTED_EDGE('',*,*,#1861,.T.);
#2489=ORIENTED_EDGE('',*,*,#1878,.T.);
#2490=ORIENTED_EDGE('',*,*,#1821,.F.);
#2491=ORIENTED_EDGE('',*,*,#1879,.T.);
#2492=ORIENTED_EDGE('',*,*,#1863,.T.);
#2493=ORIENTED_EDGE('',*,*,#1880,.T.);
#2494=ORIENTED_EDGE('',*,*,#1819,.F.);
#2495=ORIENTED_EDGE('',*,*,#1881,.T.);
#2496=ORIENTED_EDGE('',*,*,#1865,.T.);
#2497=ORIENTED_EDGE('',*,*,#1882,.T.);
#2498=ORIENTED_EDGE('',*,*,#1817,.F.);
#2499=ORIENTED_EDGE('',*,*,#1883,.T.);
#2500=ORIENTED_EDGE('',*,*,#1867,.T.);
#2501=ORIENTED_EDGE('',*,*,#1884,.T.);
#2502=ORIENTED_EDGE('',*,*,#1815,.F.);
#2503=ORIENTED_EDGE('',*,*,#1885,.T.);
#2504=ORIENTED_EDGE('',*,*,#1831,.F.);
#2505=ORIENTED_EDGE('',*,*,#1886,.T.);
#2506=ORIENTED_EDGE('',*,*,#1851,.T.);
#2507=ORIENTED_EDGE('',*,*,#1887,.T.);
#2508=ORIENTED_EDGE('',*,*,#1888,.F.);
#2509=ORIENTED_EDGE('',*,*,#1813,.F.);
#2510=ORIENTED_EDGE('',*,*,#1889,.T.);
#2511=ORIENTED_EDGE('',*,*,#1842,.T.);
#2512=ORIENTED_EDGE('',*,*,#1890,.F.);
#2513=ORIENTED_EDGE('',*,*,#1869,.T.);
#2514=ORIENTED_EDGE('',*,*,#1848,.T.);
#2515=ORIENTED_EDGE('',*,*,#1891,.F.);
#2516=ORIENTED_EDGE('',*,*,#1834,.F.);
#2517=ORIENTED_EDGE('',*,*,#1892,.T.);
#2518=ORIENTED_EDGE('',*,*,#1847,.T.);
#2519=ORIENTED_EDGE('',*,*,#1806,.F.);
#2520=ORIENTED_EDGE('',*,*,#1835,.F.);
#2521=ORIENTED_EDGE('',*,*,#1891,.T.);
#2522=ORIENTED_EDGE('',*,*,#1838,.T.);
#2523=ORIENTED_EDGE('',*,*,#1893,.T.);
#2524=ORIENTED_EDGE('',*,*,#1894,.T.);
#2525=ORIENTED_EDGE('',*,*,#1895,.F.);
#2526=ORIENTED_EDGE('',*,*,#1896,.F.);
#2527=ORIENTED_EDGE('',*,*,#1897,.T.);
#2528=ORIENTED_EDGE('',*,*,#1795,.F.);
#2529=ORIENTED_EDGE('',*,*,#1898,.T.);
#2530=ORIENTED_EDGE('',*,*,#1810,.T.);
#2531=ORIENTED_EDGE('',*,*,#1899,.F.);
#2532=ORIENTED_EDGE('',*,*,#1900,.F.);
#2533=ORIENTED_EDGE('',*,*,#1901,.T.);
#2534=ORIENTED_EDGE('',*,*,#1836,.T.);
#2535=ORIENTED_EDGE('',*,*,#1902,.T.);
#2536=ORIENTED_EDGE('',*,*,#1799,.F.);
#2537=ORIENTED_EDGE('',*,*,#1903,.T.);
#2538=ORIENTED_EDGE('',*,*,#1904,.T.);
#2539=ORIENTED_EDGE('',*,*,#1905,.T.);
#2540=ORIENTED_EDGE('',*,*,#1906,.F.);
#2541=ORIENTED_EDGE('',*,*,#1907,.T.);
#2542=ORIENTED_EDGE('',*,*,#1840,.T.);
#2543=ORIENTED_EDGE('',*,*,#1908,.T.);
#2544=ORIENTED_EDGE('',*,*,#1844,.F.);
#2545=ORIENTED_EDGE('',*,*,#1909,.F.);
#2546=ORIENTED_EDGE('',*,*,#1868,.T.);
#2547=ORIENTED_EDGE('',*,*,#1885,.F.);
#2548=ORIENTED_EDGE('',*,*,#1814,.F.);
#2549=ORIENTED_EDGE('',*,*,#1888,.T.);
#2550=ORIENTED_EDGE('',*,*,#1833,.F.);
#2551=ORIENTED_EDGE('',*,*,#1910,.T.);
#2552=ORIENTED_EDGE('',*,*,#1849,.T.);
#2553=ORIENTED_EDGE('',*,*,#1892,.F.);
#2554=ORIENTED_EDGE('',*,*,#1850,.F.);
#2555=ORIENTED_EDGE('',*,*,#1910,.F.);
#2556=ORIENTED_EDGE('',*,*,#1832,.T.);
#2557=ORIENTED_EDGE('',*,*,#1887,.F.);
#2558=ORIENTED_EDGE('',*,*,#1866,.F.);
#2559=ORIENTED_EDGE('',*,*,#1883,.F.);
#2560=ORIENTED_EDGE('',*,*,#1816,.T.);
#2561=ORIENTED_EDGE('',*,*,#1884,.F.);
#2562=ORIENTED_EDGE('',*,*,#1864,.F.);
#2563=ORIENTED_EDGE('',*,*,#1881,.F.);
#2564=ORIENTED_EDGE('',*,*,#1818,.T.);
#2565=ORIENTED_EDGE('',*,*,#1882,.F.);
#2566=ORIENTED_EDGE('',*,*,#1862,.F.);
#2567=ORIENTED_EDGE('',*,*,#1879,.F.);
#2568=ORIENTED_EDGE('',*,*,#1820,.T.);
#2569=ORIENTED_EDGE('',*,*,#1880,.F.);
#2570=ORIENTED_EDGE('',*,*,#1860,.F.);
#2571=ORIENTED_EDGE('',*,*,#1877,.F.);
#2572=ORIENTED_EDGE('',*,*,#1822,.T.);
#2573=ORIENTED_EDGE('',*,*,#1878,.F.);
#2574=ORIENTED_EDGE('',*,*,#1858,.F.);
#2575=ORIENTED_EDGE('',*,*,#1875,.F.);
#2576=ORIENTED_EDGE('',*,*,#1824,.T.);
#2577=ORIENTED_EDGE('',*,*,#1876,.F.);
#2578=ORIENTED_EDGE('',*,*,#1856,.F.);
#2579=ORIENTED_EDGE('',*,*,#1873,.F.);
#2580=ORIENTED_EDGE('',*,*,#1826,.T.);
#2581=ORIENTED_EDGE('',*,*,#1874,.F.);
#2582=ORIENTED_EDGE('',*,*,#1854,.F.);
#2583=ORIENTED_EDGE('',*,*,#1871,.F.);
#2584=ORIENTED_EDGE('',*,*,#1828,.T.);
#2585=ORIENTED_EDGE('',*,*,#1872,.F.);
#2586=ORIENTED_EDGE('',*,*,#1852,.F.);
#2587=ORIENTED_EDGE('',*,*,#1886,.F.);
#2588=ORIENTED_EDGE('',*,*,#1830,.T.);
#2589=ORIENTED_EDGE('',*,*,#1870,.F.);
#2590=ORIENTED_EDGE('',*,*,#1908,.F.);
#2591=ORIENTED_EDGE('',*,*,#1839,.T.);
#2592=ORIENTED_EDGE('',*,*,#1899,.T.);
#2593=ORIENTED_EDGE('',*,*,#1911,.F.);
#2594=ORIENTED_EDGE('',*,*,#1808,.F.);
#2595=ORIENTED_EDGE('',*,*,#1846,.T.);
#2596=ORIENTED_EDGE('',*,*,#1890,.T.);
#2597=ORIENTED_EDGE('',*,*,#1912,.F.);
#2598=ORIENTED_EDGE('',*,*,#1845,.T.);
#2599=ORIENTED_EDGE('',*,*,#1911,.T.);
#2600=ORIENTED_EDGE('',*,*,#1809,.T.);
#2601=ORIENTED_EDGE('',*,*,#1912,.T.);
#2602=ORIENTED_EDGE('',*,*,#1794,.T.);
#2603=ORIENTED_EDGE('',*,*,#1909,.T.);
#2604=ORIENTED_EDGE('',*,*,#1913,.T.);
#2605=ORIENTED_EDGE('',*,*,#1898,.F.);
#2606=ORIENTED_EDGE('',*,*,#1800,.F.);
#2607=ORIENTED_EDGE('',*,*,#1804,.T.);
#2608=ORIENTED_EDGE('',*,*,#1914,.T.);
#2609=ORIENTED_EDGE('',*,*,#1889,.F.);
#2610=ORIENTED_EDGE('',*,*,#1812,.F.);
#2611=ORIENTED_EDGE('',*,*,#1843,.F.);
#2612=ORIENTED_EDGE('',*,*,#1914,.F.);
#2613=ORIENTED_EDGE('',*,*,#1811,.F.);
#2614=ORIENTED_EDGE('',*,*,#1913,.F.);
#2615=ORIENTED_EDGE('',*,*,#1792,.T.);
#2616=ORIENTED_EDGE('',*,*,#1894,.F.);
#2617=ORIENTED_EDGE('',*,*,#1915,.T.);
#2618=ORIENTED_EDGE('',*,*,#1900,.T.);
#2619=ORIENTED_EDGE('',*,*,#1916,.T.);
#2620=ORIENTED_EDGE('',*,*,#1906,.T.);
#2621=ORIENTED_EDGE('',*,*,#1917,.F.);
#2622=ORIENTED_EDGE('',*,*,#1788,.T.);
#2623=ORIENTED_EDGE('',*,*,#1802,.F.);
#2624=ORIENTED_EDGE('',*,*,#1918,.T.);
#2625=ORIENTED_EDGE('',*,*,#1896,.T.);
#2626=ORIENTED_EDGE('',*,*,#1919,.T.);
#2627=ORIENTED_EDGE('',*,*,#1904,.F.);
#2628=ORIENTED_EDGE('',*,*,#1920,.T.);
#2629=ORIENTED_EDGE('',*,*,#1789,.F.);
#2630=ORIENTED_EDGE('',*,*,#1895,.T.);
#2631=ORIENTED_EDGE('',*,*,#1917,.T.);
#2632=ORIENTED_EDGE('',*,*,#1905,.F.);
#2633=ORIENTED_EDGE('',*,*,#1919,.F.);
#2634=ORIENTED_EDGE('',*,*,#1915,.F.);
#2635=ORIENTED_EDGE('',*,*,#1893,.F.);
#2636=ORIENTED_EDGE('',*,*,#1837,.F.);
#2637=ORIENTED_EDGE('',*,*,#1901,.F.);
#2638=ORIENTED_EDGE('',*,*,#1796,.F.);
#2639=ORIENTED_EDGE('',*,*,#1897,.F.);
#2640=ORIENTED_EDGE('',*,*,#1918,.F.);
#2641=ORIENTED_EDGE('',*,*,#1801,.F.);
#2642=ORIENTED_EDGE('',*,*,#1798,.F.);
#2643=ORIENTED_EDGE('',*,*,#1803,.F.);
#2644=ORIENTED_EDGE('',*,*,#1920,.F.);
#2645=ORIENTED_EDGE('',*,*,#1903,.F.);
#2646=ORIENTED_EDGE('',*,*,#1916,.F.);
#2647=ORIENTED_EDGE('',*,*,#1902,.F.);
#2648=ORIENTED_EDGE('',*,*,#1841,.F.);
#2649=ORIENTED_EDGE('',*,*,#1907,.F.);
#3045=CYLINDRICAL_SURFACE('',#3438,2.);
#3046=CYLINDRICAL_SURFACE('',#3441,2.);
#3047=CYLINDRICAL_SURFACE('',#3444,2.);
#3048=CYLINDRICAL_SURFACE('',#3493,1.);
#3049=CYLINDRICAL_SURFACE('',#3494,1.);
#3050=CYLINDRICAL_SURFACE('',#3495,1.);
#3051=CYLINDRICAL_SURFACE('',#3496,1.);
#3052=CYLINDRICAL_SURFACE('',#3497,1.);
#3053=CYLINDRICAL_SURFACE('',#3498,1.);
#3054=CYLINDRICAL_SURFACE('',#3499,1.);
#3055=CYLINDRICAL_SURFACE('',#3500,1.);
#3056=CYLINDRICAL_SURFACE('',#3501,1.);
#3057=CYLINDRICAL_SURFACE('',#3515,3.5);
#3058=CYLINDRICAL_SURFACE('',#3516,3.5);
#3059=CYLINDRICAL_SURFACE('',#3517,3.5);
#3060=CYLINDRICAL_SURFACE('',#3518,3.5);
#3138=ADVANCED_FACE('',(#289),#3045,.F.);
#3139=ADVANCED_FACE('',(#290),#3046,.F.);
#3140=ADVANCED_FACE('',(#291),#3047,.F.);
#3141=ADVANCED_FACE('',(#292,#121),#167,.F.);
#3142=ADVANCED_FACE('',(#293),#168,.F.);
#3143=ADVANCED_FACE('',(#294),#169,.F.);
#3144=ADVANCED_FACE('',(#295),#170,.F.);
#3145=ADVANCED_FACE('',(#296,#122),#171,.T.);
#3146=ADVANCED_FACE('',(#297),#172,.F.);
#3147=ADVANCED_FACE('',(#298),#173,.T.);
#3148=ADVANCED_FACE('',(#299),#174,.F.);
#3149=ADVANCED_FACE('',(#300),#175,.F.);
#3150=ADVANCED_FACE('',(#301),#176,.F.);
#3151=ADVANCED_FACE('',(#302),#177,.F.);
#3152=ADVANCED_FACE('',(#303),#178,.F.);
#3153=ADVANCED_FACE('',(#304),#179,.F.);
#3154=ADVANCED_FACE('',(#305),#180,.F.);
#3155=ADVANCED_FACE('',(#306),#181,.F.);
#3156=ADVANCED_FACE('',(#307),#182,.F.);
#3157=ADVANCED_FACE('',(#308),#183,.F.);
#3158=ADVANCED_FACE('',(#309),#184,.F.);
#3159=ADVANCED_FACE('',(#310),#185,.F.);
#3160=ADVANCED_FACE('',(#311),#186,.F.);
#3161=ADVANCED_FACE('',(#312),#187,.F.);
#3162=ADVANCED_FACE('',(#313),#188,.F.);
#3163=ADVANCED_FACE('',(#314),#189,.F.);
#3164=ADVANCED_FACE('',(#315),#190,.F.);
#3165=ADVANCED_FACE('',(#316),#3048,.F.);
#3166=ADVANCED_FACE('',(#317),#3049,.F.);
#3167=ADVANCED_FACE('',(#318),#3050,.F.);
#3168=ADVANCED_FACE('',(#319),#3051,.F.);
#3169=ADVANCED_FACE('',(#320),#3052,.F.);
#3170=ADVANCED_FACE('',(#321),#3053,.F.);
#3171=ADVANCED_FACE('',(#322),#3054,.F.);
#3172=ADVANCED_FACE('',(#323),#3055,.F.);
#3173=ADVANCED_FACE('',(#324),#3056,.F.);
#3174=ADVANCED_FACE('',(#325),#191,.T.);
#3175=ADVANCED_FACE('',(#326),#192,.T.);
#3176=ADVANCED_FACE('',(#327,#123),#193,.F.);
#3177=ADVANCED_FACE('',(#328),#194,.T.);
#3178=ADVANCED_FACE('',(#329),#195,.T.);
#3179=ADVANCED_FACE('',(#330,#124),#196,.F.);
#3180=ADVANCED_FACE('',(#331,#125),#197,.F.);
#3181=ADVANCED_FACE('',(#332,#126),#198,.T.);
#3182=ADVANCED_FACE('',(#333),#199,.T.);
#3183=ADVANCED_FACE('',(#334),#3057,.T.);
#3184=ADVANCED_FACE('',(#335),#3058,.T.);
#3185=ADVANCED_FACE('',(#336),#3059,.T.);
#3186=ADVANCED_FACE('',(#337),#3060,.T.);
#3270=CLOSED_SHELL('',(#3138,#3139,#3140,#3141,#3142,#3143,#3144,#3145,
#3146,#3147,#3148,#3149,#3150,#3151,#3152,#3153,#3154,#3155,#3156,#3157,
#3158,#3159,#3160,#3161,#3162,#3163,#3164,#3165,#3166,#3167,#3168,#3169,
#3170,#3171,#3172,#3173,#3174,#3175,#3176,#3177,#3178,#3179,#3180,#3181,
#3182,#3183,#3184,#3185,#3186));
#3437=AXIS2_PLACEMENT_3D('',#4922,#3952,#3953);
#3438=AXIS2_PLACEMENT_3D('',#4923,#3954,#3955);
#3439=AXIS2_PLACEMENT_3D('',#4925,#3956,#3957);
#3440=AXIS2_PLACEMENT_3D('',#4928,#3959,#3960);
#3441=AXIS2_PLACEMENT_3D('',#4929,#3961,#3962);
#3442=AXIS2_PLACEMENT_3D('',#4931,#3963,#3964);
#3443=AXIS2_PLACEMENT_3D('',#4934,#3966,#3967);
#3444=AXIS2_PLACEMENT_3D('',#4935,#3968,#3969);
#3445=AXIS2_PLACEMENT_3D('',#4937,#3970,#3971);
#3446=AXIS2_PLACEMENT_3D('',#4940,#3973,#3974);
#3447=AXIS2_PLACEMENT_3D('',#4941,#3975,#3976);
#3448=AXIS2_PLACEMENT_3D('',#4946,#3978,#3979);
#3449=AXIS2_PLACEMENT_3D('',#4950,#3981,#3982);
#3450=AXIS2_PLACEMENT_3D('',#4954,#3985,#3986);
#3451=AXIS2_PLACEMENT_3D('',#4960,#3990,#3991);
#3452=AXIS2_PLACEMENT_3D('',#4977,#4000,#4001);
#3453=AXIS2_PLACEMENT_3D('',#4987,#4006,#4007);
#3454=AXIS2_PLACEMENT_3D('',#4991,#4009,#4010);
#3455=AXIS2_PLACEMENT_3D('',#4995,#4012,#4013);
#3456=AXIS2_PLACEMENT_3D('',#4999,#4015,#4016);
#3457=AXIS2_PLACEMENT_3D('',#5003,#4018,#4019);
#3458=AXIS2_PLACEMENT_3D('',#5007,#4021,#4022);
#3459=AXIS2_PLACEMENT_3D('',#5011,#4024,#4025);
#3460=AXIS2_PLACEMENT_3D('',#5015,#4027,#4028);
#3461=AXIS2_PLACEMENT_3D('',#5019,#4030,#4031);
#3462=AXIS2_PLACEMENT_3D('',#5025,#4035,#4036);
#3463=AXIS2_PLACEMENT_3D('',#5030,#4038,#4039);
#3464=AXIS2_PLACEMENT_3D('',#5037,#4043,#4044);
#3465=AXIS2_PLACEMENT_3D('',#5038,#4045,#4046);
#3466=AXIS2_PLACEMENT_3D('',#5047,#4051,#4052);
#3467=AXIS2_PLACEMENT_3D('',#5057,#4057,#4058);
#3468=AXIS2_PLACEMENT_3D('',#5061,#4060,#4061);
#3469=AXIS2_PLACEMENT_3D('',#5065,#4063,#4064);
#3470=AXIS2_PLACEMENT_3D('',#5069,#4066,#4067);
#3471=AXIS2_PLACEMENT_3D('',#5073,#4069,#4070);
#3472=AXIS2_PLACEMENT_3D('',#5077,#4072,#4073);
#3473=AXIS2_PLACEMENT_3D('',#5081,#4075,#4076);
#3474=AXIS2_PLACEMENT_3D('',#5085,#4078,#4079);
#3475=AXIS2_PLACEMENT_3D('',#5089,#4081,#4082);
#3476=AXIS2_PLACEMENT_3D('',#5095,#4086,#4087);
#3477=AXIS2_PLACEMENT_3D('',#5098,#4090,#4091);
#3478=AXIS2_PLACEMENT_3D('',#5101,#4094,#4095);
#3479=AXIS2_PLACEMENT_3D('',#5104,#4098,#4099);
#3480=AXIS2_PLACEMENT_3D('',#5107,#4102,#4103);
#3481=AXIS2_PLACEMENT_3D('',#5110,#4106,#4107);
#3482=AXIS2_PLACEMENT_3D('',#5113,#4110,#4111);
#3483=AXIS2_PLACEMENT_3D('',#5116,#4114,#4115);
#3484=AXIS2_PLACEMENT_3D('',#5119,#4118,#4119);
#3485=AXIS2_PLACEMENT_3D('',#5122,#4122,#4123);
#3486=AXIS2_PLACEMENT_3D('',#5126,#4127,#4128);
#3487=AXIS2_PLACEMENT_3D('',#5129,#4131,#4132);
#3488=AXIS2_PLACEMENT_3D('',#5130,#4133,#4134);
#3489=AXIS2_PLACEMENT_3D('',#5142,#4142,#4143);
#3490=AXIS2_PLACEMENT_3D('',#5148,#4147,#4148);
#3491=AXIS2_PLACEMENT_3D('',#5160,#4156,#4157);
#3492=AXIS2_PLACEMENT_3D('',#5161,#4158,#4159);
#3493=AXIS2_PLACEMENT_3D('',#5163,#4161,#4162);
#3494=AXIS2_PLACEMENT_3D('',#5164,#4163,#4164);
#3495=AXIS2_PLACEMENT_3D('',#5165,#4165,#4166);
#3496=AXIS2_PLACEMENT_3D('',#5166,#4167,#4168);
#3497=AXIS2_PLACEMENT_3D('',#5167,#4169,#4170);
#3498=AXIS2_PLACEMENT_3D('',#5168,#4171,#4172);
#3499=AXIS2_PLACEMENT_3D('',#5169,#4173,#4174);
#3500=AXIS2_PLACEMENT_3D('',#5170,#4175,#4176);
#3501=AXIS2_PLACEMENT_3D('',#5171,#4177,#4178);
#3502=AXIS2_PLACEMENT_3D('',#5172,#4179,#4180);
#3503=AXIS2_PLACEMENT_3D('',#5174,#4182,#4183);
#3504=AXIS2_PLACEMENT_3D('',#5176,#4185,#4186);
#3505=AXIS2_PLACEMENT_3D('',#5177,#4187,#4188);
#3506=AXIS2_PLACEMENT_3D('',#5179,#4190,#4191);
#3507=AXIS2_PLACEMENT_3D('',#5181,#4193,#4194);
#3508=AXIS2_PLACEMENT_3D('',#5182,#4195,#4196);
#3509=AXIS2_PLACEMENT_3D('',#5183,#4197,#4198);
#3510=AXIS2_PLACEMENT_3D('',#5184,#4199,#4200);
#3511=AXIS2_PLACEMENT_3D('',#5186,#4202,#4203);
#3512=AXIS2_PLACEMENT_3D('',#5187,#4204,#4205);
#3513=AXIS2_PLACEMENT_3D('',#5189,#4207,#4208);
#3514=AXIS2_PLACEMENT_3D('',#5190,#4209,#4210);
#3515=AXIS2_PLACEMENT_3D('',#5191,#4211,#4212);
#3516=AXIS2_PLACEMENT_3D('',#5192,#4213,#4214);
#3517=AXIS2_PLACEMENT_3D('',#5193,#4215,#4216);
#3518=AXIS2_PLACEMENT_3D('',#5194,#4217,#4218);
#3952=DIRECTION('axis',(0.,0.,1.));
#3953=DIRECTION('refdir',(1.,0.,0.));
#3954=DIRECTION('center_axis',(0.,0.,1.));
#3955=DIRECTION('ref_axis',(1.,0.,0.));
#3956=DIRECTION('center_axis',(0.,0.,1.));
#3957=DIRECTION('ref_axis',(1.,0.,0.));
#3958=DIRECTION('',(0.,0.,1.));
#3959=DIRECTION('center_axis',(-2.10053591606567E-33,2.47817639425258E-17,
-1.));
#3960=DIRECTION('ref_axis',(5.20549852247368E-50,1.,2.47817639425258E-17));
#3961=DIRECTION('center_axis',(0.,0.,1.));
#3962=DIRECTION('ref_axis',(1.,0.,0.));
#3963=DIRECTION('center_axis',(-2.10053591606567E-33,2.47817639425258E-17,
-1.));
#3964=DIRECTION('ref_axis',(5.20549852247368E-50,1.,2.47817639425258E-17));
#3965=DIRECTION('',(0.,0.,1.));
#3966=DIRECTION('center_axis',(0.,0.,1.));
#3967=DIRECTION('ref_axis',(1.,0.,0.));
#3968=DIRECTION('center_axis',(5.55111512312578E-17,0.,-1.));
#3969=DIRECTION('ref_axis',(-1.,0.,-5.55111512312578E-17));
#3970=DIRECTION('center_axis',(0.,0.,-1.));
#3971=DIRECTION('ref_axis',(-1.,0.,0.));
#3972=DIRECTION('',(5.55111512312578E-17,0.,-1.));
#3973=DIRECTION('center_axis',(0.,0.,1.));
#3974=DIRECTION('ref_axis',(1.,0.,0.));
#3975=DIRECTION('center_axis',(0.,0.,-1.));
#3976=DIRECTION('ref_axis',(-1.,0.,0.));
#3977=DIRECTION('',(1.34307684565341E-16,-1.,0.));
#3978=DIRECTION('center_axis',(0.,0.,1.));
#3979=DIRECTION('ref_axis',(-1.,0.,0.));
#3980=DIRECTION('',(1.,0.,0.));
#3981=DIRECTION('center_axis',(0.,0.,1.));
#3982=DIRECTION('ref_axis',(-1.,0.,0.));
#3983=DIRECTION('',(-8.47613560090905E-17,1.,0.));
#3984=DIRECTION('',(-0.939692620785907,-0.342020143325673,0.));
#3985=DIRECTION('center_axis',(0.,1.,0.));
#3986=DIRECTION('ref_axis',(0.,0.,1.));
#3987=DIRECTION('',(0.,0.,-1.));
#3988=DIRECTION('',(1.,8.47613560090905E-17,0.));
#3989=DIRECTION('',(0.,0.,1.));
#3990=DIRECTION('center_axis',(0.766044443118972,0.642787609686546,0.));
#3991=DIRECTION('ref_axis',(-0.642787609686546,0.766044443118972,0.));
#3992=DIRECTION('',(0.,0.,-1.));
#3993=DIRECTION('',(0.642787609686546,-0.766044443118972,0.));
#3994=DIRECTION('',(0.,0.,-1.));
#3995=DIRECTION('',(0.642787609686546,-0.766044443118972,0.));
#3996=DIRECTION('',(0.,0.,1.));
#3997=DIRECTION('',(-0.642787609686546,0.766044443118972,0.));
#3998=DIRECTION('',(0.,0.,-1.));
#3999=DIRECTION('',(-0.642787609686546,0.766044443118972,0.));
#4000=DIRECTION('center_axis',(0.,0.,-1.));
#4001=DIRECTION('ref_axis',(-1.,0.,0.));
#4002=DIRECTION('',(0.766044443118972,0.642787609686546,0.));
#4003=DIRECTION('',(0.,1.,0.));
#4004=DIRECTION('',(1.,0.,0.));
#4005=DIRECTION('',(-1.23908819712629E-16,1.,0.));
#4006=DIRECTION('center_axis',(0.,0.,1.));
#4007=DIRECTION('ref_axis',(1.,0.,0.));
#4008=DIRECTION('',(-1.23908819712629E-16,1.,0.));
#4009=DIRECTION('center_axis',(0.,0.,1.));
#4010=DIRECTION('ref_axis',(1.,0.,0.));
#4011=DIRECTION('',(-1.23908819712629E-16,1.,0.));
#4012=DIRECTION('center_axis',(0.,0.,1.));
#4013=DIRECTION('ref_axis',(1.,0.,0.));
#4014=DIRECTION('',(-1.23908819712629E-16,1.,0.));
#4015=DIRECTION('center_axis',(0.,0.,1.));
#4016=DIRECTION('ref_axis',(1.,0.,0.));
#4017=DIRECTION('',(-1.23908819712629E-16,1.,0.));
#4018=DIRECTION('center_axis',(0.,0.,1.));
#4019=DIRECTION('ref_axis',(1.,0.,0.));
#4020=DIRECTION('',(-1.23908819712629E-16,1.,0.));
#4021=DIRECTION('center_axis',(0.,0.,1.));
#4022=DIRECTION('ref_axis',(1.,0.,0.));
#4023=DIRECTION('',(-1.23908819712629E-16,1.,0.));
#4024=DIRECTION('center_axis',(0.,0.,1.));
#4025=DIRECTION('ref_axis',(1.,0.,0.));
#4026=DIRECTION('',(-1.23908819712629E-16,1.,0.));
#4027=DIRECTION('center_axis',(0.,0.,1.));
#4028=DIRECTION('ref_axis',(1.,0.,0.));
#4029=DIRECTION('',(-1.23908819712629E-16,1.,0.));
#4030=DIRECTION('center_axis',(0.,0.,1.));
#4031=DIRECTION('ref_axis',(1.,0.,0.));
#4032=DIRECTION('',(-1.23908819712629E-16,1.,0.));
#4033=DIRECTION('',(-1.,0.,0.));
#4034=DIRECTION('',(-0.258819045102514,-0.96592582628907,0.));
#4035=DIRECTION('center_axis',(0.,0.,-1.));
#4036=DIRECTION('ref_axis',(-1.,0.,0.));
#4037=DIRECTION('',(1.,0.,0.));
#4038=DIRECTION('center_axis',(0.,0.,-1.));
#4039=DIRECTION('ref_axis',(-1.,0.,0.));
#4040=DIRECTION('',(1.34307684565341E-16,-1.,0.));
#4041=DIRECTION('',(-0.939692620785907,-0.342020143325673,0.));
#4042=DIRECTION('',(-8.47613560090905E-17,1.,0.));
#4043=DIRECTION('center_axis',(0.,0.,-1.));
#4044=DIRECTION('ref_axis',(-1.,0.,0.));
#4045=DIRECTION('center_axis',(-0.766044443118972,-0.642787609686546,0.));
#4046=DIRECTION('ref_axis',(0.642787609686546,-0.766044443118972,0.));
#4047=DIRECTION('',(0.,0.,-1.));
#4048=DIRECTION('',(0.642787609686547,-0.766044443118972,0.));
#4049=DIRECTION('',(0.,0.,-1.));
#4050=DIRECTION('',(0.642787609686547,-0.766044443118972,0.));
#4051=DIRECTION('center_axis',(0.,0.,-1.));
#4052=DIRECTION('ref_axis',(-1.,0.,0.));
#4053=DIRECTION('',(0.766044443118972,0.642787609686546,0.));
#4054=DIRECTION('',(-0.258819045102514,-0.96592582628907,0.));
#4055=DIRECTION('',(-1.,0.,0.));
#4056=DIRECTION('',(-1.23908819712629E-16,1.,0.));
#4057=DIRECTION('center_axis',(0.,0.,1.));
#4058=DIRECTION('ref_axis',(1.,0.,0.));
#4059=DIRECTION('',(-1.23908819712629E-16,1.,0.));
#4060=DIRECTION('center_axis',(0.,0.,1.));
#4061=DIRECTION('ref_axis',(1.,0.,0.));
#4062=DIRECTION('',(-1.23908819712629E-16,1.,0.));
#4063=DIRECTION('center_axis',(0.,0.,1.));
#4064=DIRECTION('ref_axis',(1.,0.,0.));
#4065=DIRECTION('',(-1.23908819712629E-16,1.,0.));
#4066=DIRECTION('center_axis',(0.,0.,1.));
#4067=DIRECTION('ref_axis',(1.,0.,0.));
#4068=DIRECTION('',(-1.23908819712629E-16,1.,0.));
#4069=DIRECTION('center_axis',(0.,0.,1.));
#4070=DIRECTION('ref_axis',(1.,0.,0.));
#4071=DIRECTION('',(-1.23908819712629E-16,1.,0.));
#4072=DIRECTION('center_axis',(0.,0.,1.));
#4073=DIRECTION('ref_axis',(1.,0.,0.));
#4074=DIRECTION('',(-1.23908819712629E-16,1.,0.));
#4075=DIRECTION('center_axis',(0.,0.,1.));
#4076=DIRECTION('ref_axis',(1.,0.,0.));
#4077=DIRECTION('',(-1.23908819712629E-16,1.,0.));
#4078=DIRECTION('center_axis',(0.,0.,1.));
#4079=DIRECTION('ref_axis',(1.,0.,0.));
#4080=DIRECTION('',(-1.23908819712629E-16,1.,0.));
#4081=DIRECTION('center_axis',(0.,0.,1.));
#4082=DIRECTION('ref_axis',(1.,0.,0.));
#4083=DIRECTION('',(-1.23908819712629E-16,1.,0.));
#4084=DIRECTION('',(1.,0.,0.));
#4085=DIRECTION('',(0.,1.,0.));
#4086=DIRECTION('center_axis',(-1.,-1.23908819712629E-16,0.));
#4087=DIRECTION('ref_axis',(1.23908819712629E-16,-1.,0.));
#4088=DIRECTION('',(0.,0.,1.));
#4089=DIRECTION('',(0.,0.,-1.));
#4090=DIRECTION('center_axis',(-1.,-1.23908819712629E-16,0.));
#4091=DIRECTION('ref_axis',(1.23908819712629E-16,-1.,0.));
#4092=DIRECTION('',(0.,0.,1.));
#4093=DIRECTION('',(0.,0.,-1.));
#4094=DIRECTION('center_axis',(-1.,-1.23908819712629E-16,0.));
#4095=DIRECTION('ref_axis',(1.23908819712629E-16,-1.,0.));
#4096=DIRECTION('',(0.,0.,1.));
#4097=DIRECTION('',(0.,0.,-1.));
#4098=DIRECTION('center_axis',(-1.,-1.23908819712629E-16,0.));
#4099=DIRECTION('ref_axis',(1.23908819712629E-16,-1.,0.));
#4100=DIRECTION('',(0.,0.,1.));
#4101=DIRECTION('',(0.,0.,-1.));
#4102=DIRECTION('center_axis',(-1.,-1.23908819712629E-16,0.));
#4103=DIRECTION('ref_axis',(1.23908819712629E-16,-1.,0.));
#4104=DIRECTION('',(0.,0.,1.));
#4105=DIRECTION('',(0.,0.,-1.));
#4106=DIRECTION('center_axis',(-1.,-1.23908819712629E-16,0.));
#4107=DIRECTION('ref_axis',(1.23908819712629E-16,-1.,0.));
#4108=DIRECTION('',(0.,0.,1.));
#4109=DIRECTION('',(0.,0.,-1.));
#4110=DIRECTION('center_axis',(-1.,-1.23908819712629E-16,0.));
#4111=DIRECTION('ref_axis',(1.23908819712629E-16,-1.,0.));
#4112=DIRECTION('',(0.,0.,1.));
#4113=DIRECTION('',(0.,0.,-1.));
#4114=DIRECTION('center_axis',(-1.,-1.23908819712629E-16,0.));
#4115=DIRECTION('ref_axis',(1.23908819712629E-16,-1.,0.));
#4116=DIRECTION('',(0.,0.,1.));
#4117=DIRECTION('',(0.,0.,-1.));
#4118=DIRECTION('center_axis',(-1.,-1.23908819712629E-16,0.));
#4119=DIRECTION('ref_axis',(1.23908819712629E-16,-1.,0.));
#4120=DIRECTION('',(0.,0.,-1.));
#4121=DIRECTION('',(0.,0.,1.));
#4122=DIRECTION('center_axis',(-1.,0.,0.));
#4123=DIRECTION('ref_axis',(0.,0.,1.));
#4124=DIRECTION('',(0.,0.,-1.));
#4125=DIRECTION('',(0.,0.,-1.));
#4126=DIRECTION('',(0.,0.,1.));
#4127=DIRECTION('center_axis',(0.,-1.,0.));
#4128=DIRECTION('ref_axis',(0.,0.,-1.));
#4129=DIRECTION('',(0.,0.,-1.));
#4130=DIRECTION('',(0.,0.,-1.));
#4131=DIRECTION('center_axis',(0.96592582628907,-0.258819045102514,0.));
#4132=DIRECTION('ref_axis',(0.258819045102514,0.96592582628907,0.));
#4133=DIRECTION('center_axis',(1.,1.34307684565341E-16,0.));
#4134=DIRECTION('ref_axis',(-1.34307684565341E-16,1.,0.));
#4135=DIRECTION('',(0.,0.,1.));
#4136=DIRECTION('',(-1.34307684565341E-16,1.,2.47817639425258E-17));
#4137=DIRECTION('',(0.,0.,-1.));
#4138=DIRECTION('',(-1.34307684565341E-16,1.,2.47817639425258E-17));
#4139=DIRECTION('',(0.,0.,1.));
#4140=DIRECTION('',(0.,0.,-1.));
#4141=DIRECTION('',(0.,0.,1.));
#4142=DIRECTION('center_axis',(0.,1.,0.));
#4143=DIRECTION('ref_axis',(0.,0.,1.));
#4144=DIRECTION('',(1.,8.47613560090905E-17,0.));
#4145=DIRECTION('',(0.,0.,-1.));
#4146=DIRECTION('',(0.,0.,1.));
#4147=DIRECTION('center_axis',(-1.,-8.47613560090905E-17,0.));
#4148=DIRECTION('ref_axis',(8.47613560090905E-17,-1.,0.));
#4149=DIRECTION('',(0.,0.,-1.));
#4150=DIRECTION('',(-8.47613560090905E-17,1.,2.47817639425258E-17));
#4151=DIRECTION('',(0.,0.,-1.));
#4152=DIRECTION('',(-8.47613560090905E-17,1.,2.47817639425258E-17));
#4153=DIRECTION('',(0.,0.,-1.));
#4154=DIRECTION('',(0.,0.,1.));
#4155=DIRECTION('',(0.,0.,-1.));
#4156=DIRECTION('center_axis',(0.,1.,0.));
#4157=DIRECTION('ref_axis',(0.,0.,1.));
#4158=DIRECTION('center_axis',(-1.,-1.23908819712629E-16,0.));
#4159=DIRECTION('ref_axis',(1.23908819712629E-16,-1.,0.));
#4160=DIRECTION('',(0.,0.,-1.));
#4161=DIRECTION('center_axis',(0.,0.,1.));
#4162=DIRECTION('ref_axis',(-1.,1.22464679914735E-16,0.));
#4163=DIRECTION('center_axis',(0.,0.,1.));
#4164=DIRECTION('ref_axis',(-1.,1.22464679914735E-16,0.));
#4165=DIRECTION('center_axis',(0.,0.,1.));
#4166=DIRECTION('ref_axis',(-1.,1.22464679914735E-16,0.));
#4167=DIRECTION('center_axis',(0.,0.,1.));
#4168=DIRECTION('ref_axis',(-1.,1.22464679914735E-16,0.));
#4169=DIRECTION('center_axis',(0.,0.,1.));
#4170=DIRECTION('ref_axis',(-1.,1.22464679914735E-16,0.));
#4171=DIRECTION('center_axis',(0.,0.,1.));
#4172=DIRECTION('ref_axis',(-1.,1.22464679914735E-16,0.));
#4173=DIRECTION('center_axis',(0.,0.,1.));
#4174=DIRECTION('ref_axis',(-1.,1.22464679914735E-16,0.));
#4175=DIRECTION('center_axis',(0.,0.,1.));
#4176=DIRECTION('ref_axis',(-1.,1.22464679914735E-16,0.));
#4177=DIRECTION('center_axis',(0.,0.,1.));
#4178=DIRECTION('ref_axis',(-1.,1.22464679914735E-16,0.));
#4179=DIRECTION('center_axis',(-0.342020143325673,0.939692620785907,0.));
#4180=DIRECTION('ref_axis',(-0.939692620785907,-0.342020143325673,0.));
#4181=DIRECTION('',(-0.939692620785907,-0.342020143325673,0.));
#4182=DIRECTION('center_axis',(0.642787609686546,-0.766044443118972,0.));
#4183=DIRECTION('ref_axis',(0.766044443118972,0.642787609686546,0.));
#4184=DIRECTION('',(0.766044443118972,0.642787609686546,0.));
#4185=DIRECTION('center_axis',(0.,0.,1.));
#4186=DIRECTION('ref_axis',(1.,0.,0.));
#4187=DIRECTION('center_axis',(-0.342020143325673,0.939692620785907,0.));
#4188=DIRECTION('ref_axis',(-0.939692620785907,-0.342020143325673,0.));
#4189=DIRECTION('',(-0.939692620785907,-0.342020143325673,0.));
#4190=DIRECTION('center_axis',(0.642787609686546,-0.766044443118972,0.));
#4191=DIRECTION('ref_axis',(0.766044443118972,0.642787609686546,0.));
#4192=DIRECTION('',(0.766044443118972,0.642787609686546,0.));
#4193=DIRECTION('center_axis',(0.,0.,-1.));
#4194=DIRECTION('ref_axis',(1.,0.,0.));
#4195=DIRECTION('center_axis',(-2.10053591606567E-33,2.47817639425258E-17,
-1.));
#4196=DIRECTION('ref_axis',(0.,1.,2.47817639425258E-17));
#4197=DIRECTION('center_axis',(2.10053591606567E-33,-2.47817639425258E-17,
1.));
#4198=DIRECTION('ref_axis',(5.20549852247368E-50,1.,2.47817639425258E-17));
#4199=DIRECTION('center_axis',(2.10053591606567E-33,-2.47817639425258E-17,
1.));
#4200=DIRECTION('ref_axis',(5.20549852247368E-50,1.,2.47817639425258E-17));
#4201=DIRECTION('',(1.,8.47613560090905E-17,0.));
#4202=DIRECTION('center_axis',(-2.10053591606567E-33,2.47817639425258E-17,
-1.));
#4203=DIRECTION('ref_axis',(0.,1.,2.47817639425258E-17));
#4204=DIRECTION('center_axis',(-2.10053591606567E-33,2.47817639425258E-17,
-1.));
#4205=DIRECTION('ref_axis',(5.20549852247368E-50,1.,2.47817639425258E-17));
#4206=DIRECTION('',(1.,8.47613560090905E-17,0.));
#4207=DIRECTION('center_axis',(-2.10053591606567E-33,2.47817639425258E-17,
-1.));
#4208=DIRECTION('ref_axis',(5.20549852247368E-50,1.,2.47817639425258E-17));
#4209=DIRECTION('center_axis',(8.47613560090905E-17,-1.,0.));
#4210=DIRECTION('ref_axis',(1.,8.47613560090905E-17,0.));
#4211=DIRECTION('center_axis',(0.,0.,-1.));
#4212=DIRECTION('ref_axis',(-1.,0.,0.));
#4213=DIRECTION('center_axis',(0.,0.,-1.));
#4214=DIRECTION('ref_axis',(-1.,0.,0.));
#4215=DIRECTION('center_axis',(0.,0.,-1.));
#4216=DIRECTION('ref_axis',(-1.,0.,0.));
#4217=DIRECTION('center_axis',(0.,0.,-1.));
#4218=DIRECTION('ref_axis',(-1.,0.,0.));
#4922=CARTESIAN_POINT('',(0.,0.,0.));
#4923=CARTESIAN_POINT('Origin',(26.,-116.5,-7.));
#4924=CARTESIAN_POINT('',(24.,-116.5,-7.));
#4925=CARTESIAN_POINT('Origin',(26.,-116.5,-7.));
#4926=CARTESIAN_POINT('',(24.,-116.5,-2.));
#4927=CARTESIAN_POINT('',(24.,-116.5,-7.));
#4928=CARTESIAN_POINT('Origin',(26.,-116.5,-2.));
#4929=CARTESIAN_POINT('Origin',(26.,-116.5,-7.));
#4930=CARTESIAN_POINT('',(24.,-116.5,2.));
#4931=CARTESIAN_POINT('Origin',(26.,-116.5,2.));
#4932=CARTESIAN_POINT('',(24.,-116.5,7.));
#4933=CARTESIAN_POINT('',(24.,-116.5,-7.));
#4934=CARTESIAN_POINT('Origin',(26.,-116.5,7.));
#4935=CARTESIAN_POINT('Origin',(5.,-15.2931109241333,7.));
#4936=CARTESIAN_POINT('',(7.,-15.2931109241333,5.));
#4937=CARTESIAN_POINT('Origin',(5.,-15.2931109241333,5.));
#4938=CARTESIAN_POINT('',(7.,-15.2931109241333,-5.));
#4939=CARTESIAN_POINT('',(7.,-15.2931109241333,7.));
#4940=CARTESIAN_POINT('Origin',(5.,-15.2931109241333,-5.));
#4941=CARTESIAN_POINT('Origin',(0.,0.,7.));
#4942=CARTESIAN_POINT('',(20.,-42.5037577742085,7.));
#4943=CARTESIAN_POINT('',(20.,-116.5,7.));
#4944=CARTESIAN_POINT('',(20.,-42.5037577742085,7.));
#4945=CARTESIAN_POINT('',(23.5,-120.,7.));
#4946=CARTESIAN_POINT('Origin',(23.5,-116.5,7.));
#4947=CARTESIAN_POINT('',(28.5,-120.,7.));
#4948=CARTESIAN_POINT('',(32.,-120.,7.));
#4949=CARTESIAN_POINT('',(32.,-116.5,7.));
#4950=CARTESIAN_POINT('Origin',(28.5,-116.5,7.));
#4951=CARTESIAN_POINT('',(32.,-38.136114963014,7.));
#4952=CARTESIAN_POINT('',(32.,-38.136114963014,7.));
#4953=CARTESIAN_POINT('',(20.,-42.5037577742085,7.));
#4954=CARTESIAN_POINT('Origin',(32.,-120.,7.));
#4955=CARTESIAN_POINT('',(23.5,-120.,2.));
#4956=CARTESIAN_POINT('',(23.5,-120.,7.));
#4957=CARTESIAN_POINT('',(28.5,-120.,2.));
#4958=CARTESIAN_POINT('',(-15.705120202908,-120.,2.));
#4959=CARTESIAN_POINT('',(28.5,-120.,7.));
#4960=CARTESIAN_POINT('Origin',(-15.705120202908,0.0479475016143815,7.));
#4961=CARTESIAN_POINT('',(-9.19253331742767,-7.71345131623855,7.));
#4962=CARTESIAN_POINT('',(-9.19253331742767,-7.71345131623855,5.));
#4963=CARTESIAN_POINT('',(-9.19253331742767,-7.71345131623855,7.000012));
#4964=CARTESIAN_POINT('',(-15.705120202908,0.0479475016143815,7.));
#4965=CARTESIAN_POINT('',(-15.705120202908,0.0479475016143815,7.));
#4966=CARTESIAN_POINT('',(-15.705120202908,0.0479475016143843,-7.));
#4967=CARTESIAN_POINT('',(-15.705120202908,0.0479475016143815,7.));
#4968=CARTESIAN_POINT('',(-9.19253331742767,-7.71345131623855,-7.));
#4969=CARTESIAN_POINT('',(-15.705120202908,0.0479475016143815,-7.));
#4970=CARTESIAN_POINT('',(-9.19253331742767,-7.71345131623855,-5.));
#4971=CARTESIAN_POINT('',(-9.19253331742767,-7.71345131623855,-7.000012));
#4972=CARTESIAN_POINT('',(20.,-42.5037577742085,-5.));
#4973=CARTESIAN_POINT('',(-9.19253331742767,-7.71345131623855,-5.));
#4974=CARTESIAN_POINT('',(20.,-42.5037577742085,5.));
#4975=CARTESIAN_POINT('',(20.,-42.5037577742085,7.));
#4976=CARTESIAN_POINT('',(-9.19253331742767,-7.71345131623855,5.));
#4977=CARTESIAN_POINT('Origin',(0.,0.,7.));
#4978=CARTESIAN_POINT('',(0.,0.,7.));
#4979=CARTESIAN_POINT('',(0.,0.,7.));
#4980=CARTESIAN_POINT('',(0.,5.,7.));
#4981=CARTESIAN_POINT('',(0.,0.,7.));
#4982=CARTESIAN_POINT('',(5.,5.,7.));
#4983=CARTESIAN_POINT('',(0.,5.,7.));
#4984=CARTESIAN_POINT('',(5.,9.,7.));
#4985=CARTESIAN_POINT('',(5.,40.,7.));
#4986=CARTESIAN_POINT('',(5.,11.,7.));
#4987=CARTESIAN_POINT('Origin',(5.00000000000001,10.,7.));
#4988=CARTESIAN_POINT('',(5.,12.5,7.));
#4989=CARTESIAN_POINT('',(5.,40.,7.));
#4990=CARTESIAN_POINT('',(5.,14.5,7.));
#4991=CARTESIAN_POINT('Origin',(5.00000000000001,13.5,7.));
#4992=CARTESIAN_POINT('',(5.,16.,7.));
#4993=CARTESIAN_POINT('',(5.,40.,7.));
#4994=CARTESIAN_POINT('',(5.,18.,7.));
#4995=CARTESIAN_POINT('Origin',(5.00000000000001,17.,7.));
#4996=CARTESIAN_POINT('',(5.,19.5,7.));
#4997=CARTESIAN_POINT('',(5.,40.,7.));
#4998=CARTESIAN_POINT('',(5.,21.5,7.));
#4999=CARTESIAN_POINT('Origin',(5.00000000000001,20.5,7.));
#5000=CARTESIAN_POINT('',(5.,23.,7.));
#5001=CARTESIAN_POINT('',(5.,40.,7.));
#5002=CARTESIAN_POINT('',(5.,25.,7.));
#5003=CARTESIAN_POINT('Origin',(5.00000000000001,24.,7.));
#5004=CARTESIAN_POINT('',(5.,26.5,7.));
#5005=CARTESIAN_POINT('',(5.,40.,7.));
#5006=CARTESIAN_POINT('',(5.,28.5,7.));
#5007=CARTESIAN_POINT('Origin',(5.00000000000001,27.5,7.));
#5008=CARTESIAN_POINT('',(5.,30.,7.));
#5009=CARTESIAN_POINT('',(5.,40.,7.));
#5010=CARTESIAN_POINT('',(5.,32.,7.));
#5011=CARTESIAN_POINT('Origin',(5.00000000000001,31.,7.));
#5012=CARTESIAN_POINT('',(5.,33.5,7.));
#5013=CARTESIAN_POINT('',(5.,40.,7.));
#5014=CARTESIAN_POINT('',(5.,35.5,7.));
#5015=CARTESIAN_POINT('Origin',(5.00000000000001,34.5,7.));
#5016=CARTESIAN_POINT('',(5.,37.,7.));
#5017=CARTESIAN_POINT('',(5.,40.,7.));
#5018=CARTESIAN_POINT('',(5.,39.,7.));
#5019=CARTESIAN_POINT('Origin',(5.,38.,7.));
#5020=CARTESIAN_POINT('',(5.,40.,7.));
#5021=CARTESIAN_POINT('',(5.,40.,7.));
#5022=CARTESIAN_POINT('',(-5.,40.,7.));
#5023=CARTESIAN_POINT('',(0.,40.,7.));
#5024=CARTESIAN_POINT('',(-5.,40.,7.));
#5025=CARTESIAN_POINT('Origin',(0.,0.,-7.));
#5026=CARTESIAN_POINT('',(23.5,-120.,-7.));
#5027=CARTESIAN_POINT('',(28.5,-120.,-7.));
#5028=CARTESIAN_POINT('',(32.,-120.,-7.));
#5029=CARTESIAN_POINT('',(20.,-116.5,-7.));
#5030=CARTESIAN_POINT('Origin',(23.5,-116.5,-7.));
#5031=CARTESIAN_POINT('',(20.,-42.5037577742085,-7.));
#5032=CARTESIAN_POINT('',(20.,-42.5037577742085,-7.));
#5033=CARTESIAN_POINT('',(32.,-38.136114963014,-7.));
#5034=CARTESIAN_POINT('',(20.,-42.5037577742085,-7.));
#5035=CARTESIAN_POINT('',(32.,-116.5,-7.));
#5036=CARTESIAN_POINT('',(32.,-38.136114963014,-7.));
#5037=CARTESIAN_POINT('Origin',(28.5,-116.5,-7.));
#5038=CARTESIAN_POINT('Origin',(0.,0.,7.));
#5039=CARTESIAN_POINT('',(0.,0.,5.));
#5040=CARTESIAN_POINT('',(0.,0.,-5.));
#5041=CARTESIAN_POINT('',(0.,0.,7.));
#5042=CARTESIAN_POINT('',(32.,-38.136114963014,5.));
#5043=CARTESIAN_POINT('',(32.,-38.136114963014,5.));
#5044=CARTESIAN_POINT('',(32.,-38.136114963014,-5.));
#5045=CARTESIAN_POINT('',(32.,-38.136114963014,7.));
#5046=CARTESIAN_POINT('',(32.,-38.136114963014,-5.));
#5047=CARTESIAN_POINT('Origin',(0.,0.,-7.));
#5048=CARTESIAN_POINT('',(0.,0.,-7.));
#5049=CARTESIAN_POINT('',(0.,0.,-7.));
#5050=CARTESIAN_POINT('',(-5.,40.,-7.));
#5051=CARTESIAN_POINT('',(-5.,40.,-7.));
#5052=CARTESIAN_POINT('',(5.,40.,-7.));
#5053=CARTESIAN_POINT('',(0.,40.,-7.));
#5054=CARTESIAN_POINT('',(5.,39.,-7.));
#5055=CARTESIAN_POINT('',(5.,40.,-7.));
#5056=CARTESIAN_POINT('',(5.,37.,-7.));
#5057=CARTESIAN_POINT('Origin',(5.,38.,-7.));
#5058=CARTESIAN_POINT('',(5.,35.5,-7.));
#5059=CARTESIAN_POINT('',(5.,40.,-7.));
#5060=CARTESIAN_POINT('',(5.,33.5,-7.));
#5061=CARTESIAN_POINT('Origin',(5.00000000000001,34.5,-7.));
#5062=CARTESIAN_POINT('',(5.,32.,-7.));
#5063=CARTESIAN_POINT('',(5.,40.,-7.));
#5064=CARTESIAN_POINT('',(5.,30.,-7.));
#5065=CARTESIAN_POINT('Origin',(5.00000000000001,31.,-7.));
#5066=CARTESIAN_POINT('',(5.,28.5,-7.));
#5067=CARTESIAN_POINT('',(5.,40.,-7.));
#5068=CARTESIAN_POINT('',(5.,26.5,-7.));
#5069=CARTESIAN_POINT('Origin',(5.00000000000001,27.5,-7.));
#5070=CARTESIAN_POINT('',(5.,25.,-7.));
#5071=CARTESIAN_POINT('',(5.,40.,-7.));
#5072=CARTESIAN_POINT('',(5.,23.,-7.));
#5073=CARTESIAN_POINT('Origin',(5.00000000000001,24.,-7.));
#5074=CARTESIAN_POINT('',(5.,21.5,-7.));
#5075=CARTESIAN_POINT('',(5.,40.,-7.));
#5076=CARTESIAN_POINT('',(5.,19.5,-7.));
#5077=CARTESIAN_POINT('Origin',(5.00000000000001,20.5,-7.));
#5078=CARTESIAN_POINT('',(5.,18.,-7.));
#5079=CARTESIAN_POINT('',(5.,40.,-7.));
#5080=CARTESIAN_POINT('',(5.,16.,-7.));
#5081=CARTESIAN_POINT('Origin',(5.00000000000001,17.,-7.));
#5082=CARTESIAN_POINT('',(5.,14.5,-7.));
#5083=CARTESIAN_POINT('',(5.,40.,-7.));
#5084=CARTESIAN_POINT('',(5.,12.5,-7.));
#5085=CARTESIAN_POINT('Origin',(5.00000000000001,13.5,-7.));
#5086=CARTESIAN_POINT('',(5.,11.,-7.));
#5087=CARTESIAN_POINT('',(5.,40.,-7.));
#5088=CARTESIAN_POINT('',(5.,9.,-7.));
#5089=CARTESIAN_POINT('Origin',(5.00000000000001,10.,-7.));
#5090=CARTESIAN_POINT('',(5.,5.,-7.));
#5091=CARTESIAN_POINT('',(5.,40.,-7.));
#5092=CARTESIAN_POINT('',(0.,5.,-7.));
#5093=CARTESIAN_POINT('',(0.,5.,-7.));
#5094=CARTESIAN_POINT('',(0.,0.,-7.));
#5095=CARTESIAN_POINT('Origin',(5.,40.,7.));
#5096=CARTESIAN_POINT('',(5.,33.5,-7.));
#5097=CARTESIAN_POINT('',(5.,32.,-7.));
#5098=CARTESIAN_POINT('Origin',(5.,40.,7.));
#5099=CARTESIAN_POINT('',(5.,30.,-7.));
#5100=CARTESIAN_POINT('',(5.,28.5,-7.));
#5101=CARTESIAN_POINT('Origin',(5.,40.,7.));
#5102=CARTESIAN_POINT('',(5.,26.5,-7.));
#5103=CARTESIAN_POINT('',(5.,25.,-7.));
#5104=CARTESIAN_POINT('Origin',(5.,40.,7.));
#5105=CARTESIAN_POINT('',(5.,23.,-7.));
#5106=CARTESIAN_POINT('',(5.,21.5,-7.));
#5107=CARTESIAN_POINT('Origin',(5.,40.,7.));
#5108=CARTESIAN_POINT('',(5.,19.5,-7.));
#5109=CARTESIAN_POINT('',(5.,18.,-7.));
#5110=CARTESIAN_POINT('Origin',(5.,40.,7.));
#5111=CARTESIAN_POINT('',(5.,16.,-7.));
#5112=CARTESIAN_POINT('',(5.,14.5,-7.));
#5113=CARTESIAN_POINT('Origin',(5.,40.,7.));
#5114=CARTESIAN_POINT('',(5.,12.5,-7.));
#5115=CARTESIAN_POINT('',(5.,11.,-7.));
#5116=CARTESIAN_POINT('Origin',(5.,40.,7.));
#5117=CARTESIAN_POINT('',(5.,9.,-7.));
#5118=CARTESIAN_POINT('',(5.,5.,7.));
#5119=CARTESIAN_POINT('Origin',(5.,40.,7.));
#5120=CARTESIAN_POINT('',(5.,35.5,-7.));
#5121=CARTESIAN_POINT('',(5.,37.,-7.));
#5122=CARTESIAN_POINT('Origin',(0.,0.,7.));
#5123=CARTESIAN_POINT('',(0.,5.,7.));
#5124=CARTESIAN_POINT('',(0.,0.,7.));
#5125=CARTESIAN_POINT('',(0.,0.,-7.000012));
#5126=CARTESIAN_POINT('Origin',(0.,40.,7.));
#5127=CARTESIAN_POINT('',(-5.,40.,7.));
#5128=CARTESIAN_POINT('',(5.,40.,7.));
#5129=CARTESIAN_POINT('Origin',(-5.,40.,7.));
#5130=CARTESIAN_POINT('Origin',(20.,-42.5037577742085,7.));
#5131=CARTESIAN_POINT('',(20.,-116.5,-2.));
#5132=CARTESIAN_POINT('',(20.,-116.5,7.));
#5133=CARTESIAN_POINT('',(20.,-50.,-2.));
#5134=CARTESIAN_POINT('',(20.,-42.5037577742085,-2.));
#5135=CARTESIAN_POINT('',(20.,-50.,2.));
#5136=CARTESIAN_POINT('',(20.,-50.,7.));
#5137=CARTESIAN_POINT('',(20.,-116.5,2.));
#5138=CARTESIAN_POINT('',(20.,-42.5037577742085,2.));
#5139=CARTESIAN_POINT('',(20.,-116.5,7.));
#5140=CARTESIAN_POINT('',(20.,-42.5037577742085,7.));
#5141=CARTESIAN_POINT('',(20.,-42.5037577742085,-7.000012));
#5142=CARTESIAN_POINT('Origin',(32.,-120.,7.));
#5143=CARTESIAN_POINT('',(23.5,-120.,-2.));
#5144=CARTESIAN_POINT('',(28.5,-120.,-2.));
#5145=CARTESIAN_POINT('',(-15.705120202908,-120.,-2.));
#5146=CARTESIAN_POINT('',(23.5,-120.,7.));
#5147=CARTESIAN_POINT('',(28.5,-120.,7.));
#5148=CARTESIAN_POINT('Origin',(32.,-38.136114963014,7.));
#5149=CARTESIAN_POINT('',(32.,-116.5,2.));
#5150=CARTESIAN_POINT('',(32.,-116.5,7.));
#5151=CARTESIAN_POINT('',(32.,-50.,2.));
#5152=CARTESIAN_POINT('',(32.,-120.,2.));
#5153=CARTESIAN_POINT('',(32.,-50.,-2.));
#5154=CARTESIAN_POINT('',(32.,-50.,2.));
#5155=CARTESIAN_POINT('',(32.,-116.5,-2.));
#5156=CARTESIAN_POINT('',(32.,-120.,-2.));
#5157=CARTESIAN_POINT('',(32.,-116.5,7.));
#5158=CARTESIAN_POINT('',(32.,-38.136114963014,-7.000012));
#5159=CARTESIAN_POINT('',(32.,-38.136114963014,7.));
#5160=CARTESIAN_POINT('Origin',(0.,5.,7.));
#5161=CARTESIAN_POINT('Origin',(5.,40.,7.));
#5162=CARTESIAN_POINT('',(5.,39.,-7.));
#5163=CARTESIAN_POINT('Origin',(5.,38.,-7.));
#5164=CARTESIAN_POINT('Origin',(5.00000000000001,10.,-7.));
#5165=CARTESIAN_POINT('Origin',(5.00000000000001,13.5,-7.));
#5166=CARTESIAN_POINT('Origin',(5.00000000000001,17.,-7.));
#5167=CARTESIAN_POINT('Origin',(5.00000000000001,20.5,-7.));
#5168=CARTESIAN_POINT('Origin',(5.00000000000001,24.,-7.));
#5169=CARTESIAN_POINT('Origin',(5.00000000000001,27.5,-7.));
#5170=CARTESIAN_POINT('Origin',(5.00000000000001,31.,-7.));
#5171=CARTESIAN_POINT('Origin',(5.00000000000001,34.5,-7.));
#5172=CARTESIAN_POINT('Origin',(20.,-42.5037577742085,-7.000012));
#5173=CARTESIAN_POINT('',(20.,-42.5037577742085,-5.));
#5174=CARTESIAN_POINT('Origin',(0.,0.,-7.000012));
#5175=CARTESIAN_POINT('',(0.,0.,-5.));
#5176=CARTESIAN_POINT('Origin',(0.,0.,-5.));
#5177=CARTESIAN_POINT('Origin',(20.,-42.5037577742085,7.000012));
#5178=CARTESIAN_POINT('',(20.,-42.5037577742085,5.));
#5179=CARTESIAN_POINT('Origin',(0.,0.,7.000012));
#5180=CARTESIAN_POINT('',(0.,0.,5.));
#5181=CARTESIAN_POINT('Origin',(0.,0.,5.));
#5182=CARTESIAN_POINT('Origin',(-15.705120202908,-120.,-2.));
#5183=CARTESIAN_POINT('Origin',(23.5,-116.5,-2.));
#5184=CARTESIAN_POINT('Origin',(28.5,-116.5,-2.));
#5185=CARTESIAN_POINT('',(-15.705120202908,-50.,-2.));
#5186=CARTESIAN_POINT('Origin',(-15.705120202908,-120.,2.));
#5187=CARTESIAN_POINT('Origin',(23.5,-116.5,2.));
#5188=CARTESIAN_POINT('',(-15.705120202908,-50.,2.));
#5189=CARTESIAN_POINT('Origin',(28.5,-116.5,2.));
#5190=CARTESIAN_POINT('Origin',(-15.705120202908,-50.,2.));
#5191=CARTESIAN_POINT('Origin',(23.5,-116.5,7.));
#5192=CARTESIAN_POINT('Origin',(23.5,-116.5,7.));
#5193=CARTESIAN_POINT('Origin',(28.5,-116.5,7.));
#5194=CARTESIAN_POINT('Origin',(28.5,-116.5,7.));
#5975=UNCERTAINTY_MEASURE_WITH_UNIT(LENGTH_MEASURE(0.01),#5991,
'DISTANCE_ACCURACY_VALUE',
'Maximum model space distance between geometric entities at asserted c
onnectivities');
#5981=UNCERTAINTY_MEASURE_WITH_UNIT(LENGTH_MEASURE(0.01),#5991,
'DISTANCE_ACCURACY_VALUE',
'Maximum model space distance between geometric entities at asserted c
onnectivities');
#5984=(
GEOMETRIC_REPRESENTATION_CONTEXT(3)
GLOBAL_UNCERTAINTY_ASSIGNED_CONTEXT((#5975))
GLOBAL_UNIT_ASSIGNED_CONTEXT((#5991,#5993,#5994))
REPRESENTATION_CONTEXT('','3D')
);
#5990=(
GEOMETRIC_REPRESENTATION_CONTEXT(3)
GLOBAL_UNCERTAINTY_ASSIGNED_CONTEXT((#5981))
GLOBAL_UNIT_ASSIGNED_CONTEXT((#5991,#5993,#5994))
REPRESENTATION_CONTEXT('','3D')
);
#5991=(
LENGTH_UNIT()
NAMED_UNIT(*)
SI_UNIT(.MILLI.,.METRE.)
);
#5993=(
NAMED_UNIT(*)
PLANE_ANGLE_UNIT()
SI_UNIT($,.RADIAN.)
);
#5994=(
NAMED_UNIT(*)
SI_UNIT($,.STERADIAN.)
SOLID_ANGLE_UNIT()
);
#5997=SHAPE_DEFINITION_REPRESENTATION(#6005,#6022);
#6005=PRODUCT_DEFINITION_SHAPE('',$,#6031);
#6022=SHAPE_REPRESENTATION('',(#3437),#5984);
#6028=PRODUCT_DEFINITION_CONTEXT('part definition',#6054,'design');
#6031=PRODUCT_DEFINITION('Pliers Jaw 2','Pliers Jaw 2',#6039,#6028);
#6039=PRODUCT_DEFINITION_FORMATION('',$,#6058);
#6054=APPLICATION_CONTEXT(
'Core Data for Automotive Mechanical Design Process');
#6055=PRODUCT_CONTEXT('part definition',#6054,'mechanical');
#6058=PRODUCT('Pliers Jaw 2','Pliers Jaw 2',$,(#6055));
#6065=PRESENTATION_STYLE_ASSIGNMENT((#6071));
#6071=SURFACE_STYLE_USAGE(.BOTH.,#6077);
#6077=SURFACE_SIDE_STYLE('',(#6083));
#6083=SURFACE_STYLE_FILL_AREA(#6089);
#6089=FILL_AREA_STYLE('Opaque(61,176,222)',(#6095));
#6095=FILL_AREA_STYLE_COLOUR('Opaque(61,176,222)',#6101);
#6101=COLOUR_RGB('Opaque(61,176,222)',0.23921568627451,0.690196078431373,
0.870588235294118);
ENDSEC;
END-ISO-10303-21;
